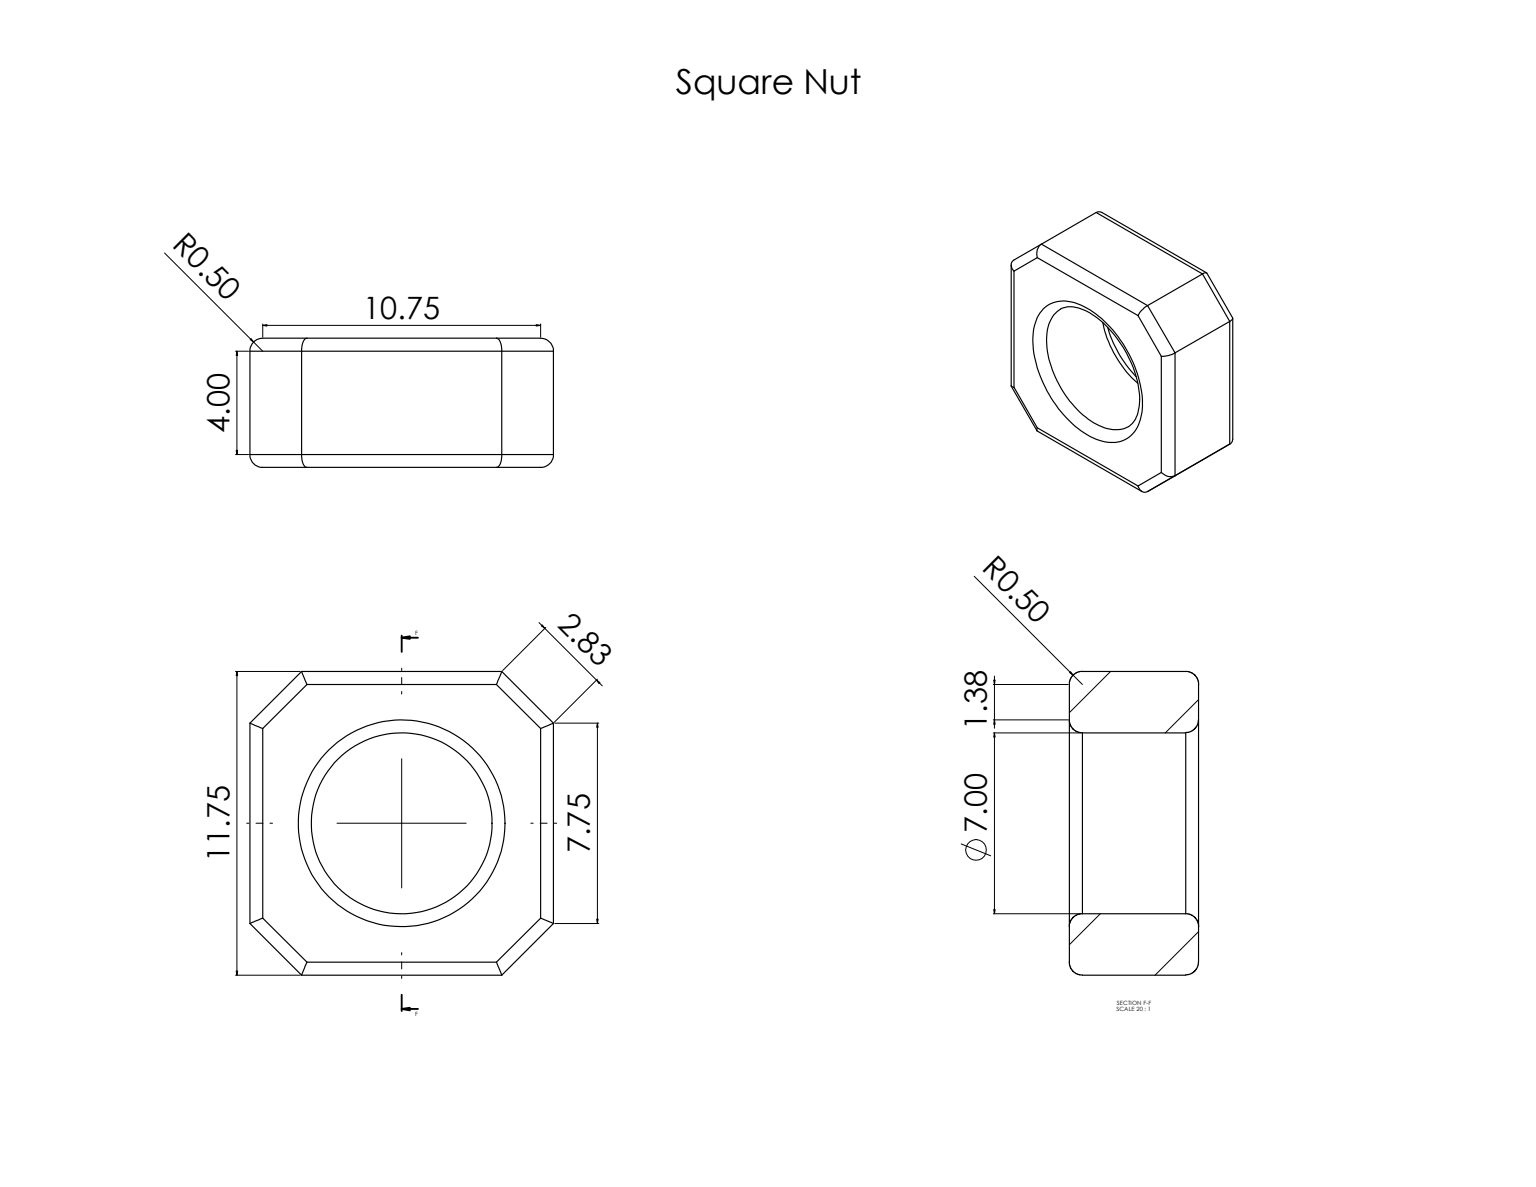
ISO-10303-21;
HEADER;
FILE_DESCRIPTION (('STEP AP214'),
    '1' );
FILE_NAME ('Square Nut.step',
    '2026-10-25T21:42:00',
    ( '' ),
    ( '' ),
    'SwSTEP 2.0',
    'SolidWorks 2025',
    '' );
FILE_SCHEMA (( 'AUTOMOTIVE_DESIGN' ));
ENDSEC;

DATA;
#32=VECTOR ( 'NONE', #10957, 1000.000000000000000 ) ;
#147=EDGE_LOOP ( 'NONE', ( #29391, #20938, #24659, #15667, #28706, #3873, #20369, #28509 ) ) ;
#209=ORIENTED_EDGE ( 'NONE', *, *, #21676, .F. ) ;
#298=LINE ( 'NONE', #12862, #20525 ) ;
#314=ORIENTED_EDGE ( 'NONE', *, *, #36050, .T. ) ;
#343=VECTOR ( 'NONE', #5203, 999.9999999999998863 ) ;
#423=ORIENTED_EDGE ( 'NONE', *, *, #22211, .T. ) ;
#429=CARTESIAN_POINT ( 'NONE',  ( 0.000000000000000000, 17.49999999999998934, -84.65254291642213502 ) ) ;
#439=EDGE_CURVE ( 'NONE', #4506, #37991, #39370, .T. ) ;
#451=( NAMED_UNIT ( * ) PLANE_ANGLE_UNIT ( ) SI_UNIT ( $, .RADIAN. ) );
#460=DIRECTION ( 'NONE',  ( 1.000000000000000000, 0.000000000000000000, 0.000000000000000000 ) ) ;
#514=EDGE_CURVE ( 'NONE', #7458, #11015, #14082, .T. ) ;
#541=ADVANCED_FACE ( 'NONE', ( #26216 ), #32999, .F. ) ;
#599=VECTOR ( 'NONE', #23370, 1000.000000000000000 ) ;
#676=AXIS2_PLACEMENT_3D ( 'NONE', #31077, #40644, #5545 ) ;
#731=CYLINDRICAL_SURFACE ( 'NONE', #34237, 0.5000000000000004441 ) ;
#739=ADVANCED_FACE ( 'NONE', ( #24084 ), #20878, .T. ) ;
#747=DIRECTION ( 'NONE',  ( 0.000000000000000000, -0.000000000000000000, 1.000000000000000000 ) ) ;
#835=AXIS2_PLACEMENT_3D ( 'NONE', #18209, #14814, #11404 ) ;
#865=ORIENTED_EDGE ( 'NONE', *, *, #17748, .T. ) ;
#951=PLANE ( 'NONE',  #3002 ) ;
#1004=ORIENTED_EDGE ( 'NONE', *, *, #3760, .F. ) ;
#1026=DIRECTION ( 'NONE',  ( 0.000000000000000000, 0.000000000000000000, -1.000000000000000000 ) ) ;
#1027=DIRECTION ( 'NONE',  ( -0.7071067811865469066, -0.7071067811865482389, -0.000000000000000000 ) ) ;
#1093=PLANE ( 'NONE',  #33638 ) ;
#1147=EDGE_CURVE ( 'NONE', #19379, #7458, #41009, .T. ) ;
#1148=DIRECTION ( 'NONE',  ( 0.000000000000000000, -0.000000000000000000, 1.000000000000000000 ) ) ;
#1215=CYLINDRICAL_SURFACE ( 'NONE', #6156, 0.5000000000000004441 ) ;
#1238=CYLINDRICAL_SURFACE ( 'NONE', #24874, 0.5000000000000006661 ) ;
#1268=DIRECTION ( 'NONE',  ( 0.000000000000000000, -0.000000000000000000, 1.000000000000000000 ) ) ;
#1309=CARTESIAN_POINT ( 'NONE',  ( 5.876432148649220366, 13.62356785135077075, -80.65254291642212081 ) ) ;
#1364=ORIENTED_EDGE ( 'NONE', *, *, #11107, .F. ) ;
#1384=CARTESIAN_POINT ( 'NONE',  ( -3.876432148649210152, 11.62356785135076542, -85.15254291642213502 ) ) ;
#1493=ORIENTED_EDGE ( 'NONE', *, *, #11107, .T. ) ;
#1543=ADVANCED_FACE ( 'NONE', ( #16227 ), #29170, .F. ) ;
#1548=ORIENTED_EDGE ( 'NONE', *, *, #4783, .F. ) ;
#1552=( LENGTH_UNIT ( ) NAMED_UNIT ( * ) SI_UNIT ( .MILLI., .METRE. ) );
#1590=EDGE_LOOP ( 'NONE', ( #18017, #2676, #21565, #27525 ) ) ;
#1591=CARTESIAN_POINT ( 'NONE',  ( -3.669325367462682230, 22.87643214864920438, -85.15254291642213502 ) ) ;
#1626=DIRECTION ( 'NONE',  ( 0.000000000000000000, -1.000000000000000000, 0.000000000000000000 ) ) ;
#1760=AXIS2_PLACEMENT_3D ( 'NONE', #429, #40567, #7833 ) ;
#1873=CARTESIAN_POINT ( 'NONE',  ( 0.000000000000000000, 17.49999999999998934, -84.65254291642213502 ) ) ;
#1918=CARTESIAN_POINT ( 'NONE',  ( -4.227121241944041152, 4.227121241944031382, -84.65254291642213502 ) ) ;
#1965=CARTESIAN_POINT ( 'NONE',  ( 5.876432148649220366, 13.62356785135077075, -84.65254291642213502 ) ) ;
#1990=ORIENTED_EDGE ( 'NONE', *, *, #41545, .T. ) ;
#1995=( BOUNDED_CURVE ( )  B_SPLINE_CURVE ( 3, ( #10609, #7625, #33578, #29950 ),
 .UNSPECIFIED., .F., .T. ) 
 B_SPLINE_CURVE_WITH_KNOTS ( ( 4, 4 ),
 ( 4.712388980384687009, 6.283185307179586232 ),
 .UNSPECIFIED. ) 
 CURVE ( )  GEOMETRIC_REPRESENTATION_ITEM ( )  RATIONAL_B_SPLINE_CURVE ( ( 1.000000000000000000, 0.8047378541243643824, 0.8047378541243643824, 1.000000000000000000 ) ) 
 REPRESENTATION_ITEM ( '' )  );
#1996=ORIENTED_EDGE ( 'NONE', *, *, #24896, .F. ) ;
#2058=VECTOR ( 'NONE', #38392, 1000.000000000000114 ) ;
#2077=CARTESIAN_POINT ( 'NONE',  ( -3.876432148649222142, 23.37643214864920438, -84.65254291642213502 ) ) ;
#2139=ORIENTED_EDGE ( 'NONE', *, *, #24461, .F. ) ;
#2181=DIRECTION ( 'NONE',  ( -0.7071067811865491270, 0.7071067811865460184, 0.000000000000000000 ) ) ;
#2237=CARTESIAN_POINT ( 'NONE',  ( 5.876432148649220366, 21.37643214864921148, -84.65254291642213502 ) ) ;
#2249=FACE_OUTER_BOUND ( 'NONE', #36965, .T. ) ;
#2266=CARTESIAN_POINT ( 'NONE',  ( 3.876432148649220366, 11.62356785135076542, -80.65254291642212081 ) ) ;
#2363=EDGE_LOOP ( 'NONE', ( #33667, #25250 ) ) ;
#2397=TOROIDAL_SURFACE ( 'NONE', #13937, 4.000000000000003553, 0.5000000000000000000 ) ;
#2455=VERTEX_POINT ( 'NONE', #23151 ) ;
#2474=ORIENTED_EDGE ( 'NONE', *, *, #36963, .T. ) ;
#2499=FACE_OUTER_BOUND ( 'NONE', #41086, .T. ) ;
#2517=ADVANCED_FACE ( 'NONE', ( #16367 ), #9981, .F. ) ;
#2561=ORIENTED_EDGE ( 'NONE', *, *, #32470, .T. ) ;
#2601=ORIENTED_EDGE ( 'NONE', *, *, #36050, .F. ) ;
#2676=ORIENTED_EDGE ( 'NONE', *, *, #13612, .F. ) ;
#2698=AXIS2_PLACEMENT_3D ( 'NONE', #15484, #25686, #38648 ) ;
#2718=DIRECTION ( 'NONE',  ( -0.7071067811865465735, -0.7071067811865483499, -0.000000000000000000 ) ) ;
#2762=DIRECTION ( 'NONE',  ( 0.7071067811865490160, -0.7071067811865460184, -0.000000000000000000 ) ) ;
#2811=DIRECTION ( 'NONE',  ( 0.000000000000000000, 0.000000000000000000, -1.000000000000000000 ) ) ;
#2845=EDGE_CURVE ( 'NONE', #19607, #21730, #21811, .T. ) ;
#2917=CARTESIAN_POINT ( 'NONE',  ( 3.669325367462673793, 12.12356785135076542, -80.15254291642212081 ) ) ;
#2983=ORIENTED_EDGE ( 'NONE', *, *, #7409, .T. ) ;
#3002=AXIS2_PLACEMENT_3D ( 'NONE', #30076, #23711, #13917 ) ;
#3094=ADVANCED_FACE ( 'NONE', ( #32468 ), #36285, .T. ) ;
#3161=ORIENTED_EDGE ( 'NONE', *, *, #23680, .T. ) ;
#3163=VECTOR ( 'NONE', #21410, 1000.000000000000000 ) ;
#3352=DIRECTION ( 'NONE',  ( -1.000000000000000000, -0.000000000000000000, -0.000000000000000000 ) ) ;
#3399=ORIENTED_EDGE ( 'NONE', *, *, #5823, .T. ) ;
#3527=DIRECTION ( 'NONE',  ( 1.000000000000000000, 0.000000000000000000, -0.000000000000000000 ) ) ;
#3569=AXIS2_PLACEMENT_3D ( 'NONE', #31939, #13418, #2811 ) ;
#3608=ADVANCED_FACE ( 'NONE', ( #17255 ), #1093, .F. ) ;
#3668=VERTEX_POINT ( 'NONE', #26610 ) ;
#3679=AXIS2_PLACEMENT_3D ( 'NONE', #26780, #39745, #29310 ) ;
#3745=CARTESIAN_POINT ( 'NONE',  ( -4.227121241944041152, 4.227121241944031382, -80.65254291642212081 ) ) ;
#3760=EDGE_CURVE ( 'NONE', #27278, #9802, #11736, .T. ) ;
#3765=CARTESIAN_POINT ( 'NONE',  ( -5.876432148649216813, 13.62356785135076365, -80.35964969760868826 ) ) ;
#3777=AXIS2_PLACEMENT_3D ( 'NONE', #10554, #23535, #36496 ) ;
#3816=CARTESIAN_POINT ( 'NONE',  ( 5.376432148649220366, 11.62356785135076542, -80.65254291642212081 ) ) ;
#3840=ORIENTED_EDGE ( 'NONE', *, *, #23636, .T. ) ;
#3856=DIRECTION ( 'NONE',  ( 1.000000000000000000, 0.000000000000000000, 0.000000000000000000 ) ) ;
#3873=ORIENTED_EDGE ( 'NONE', *, *, #4783, .T. ) ;
#3931=EDGE_LOOP ( 'NONE', ( #11008, #40649, #40449, #39510 ) ) ;
#4095=CARTESIAN_POINT ( 'NONE',  ( -5.669325367462669796, 13.70935428897766428, -85.15254291642212081 ) ) ;
#4249=AXIS2_PLACEMENT_3D ( 'NONE', #22294, #5923, #12518 ) ;
#4280=CARTESIAN_POINT ( 'NONE',  ( 0.000000000000000000, 17.49999999999998934, -80.65254291642212081 ) ) ;
#4479=ORIENTED_EDGE ( 'NONE', *, *, #27721, .F. ) ;
#4506=VERTEX_POINT ( 'NONE', #29675 ) ;
#4555=CYLINDRICAL_SURFACE ( 'NONE', #36145, 0.5000000000000000000 ) ;
#4624=VERTEX_POINT ( 'NONE', #17969 ) ;
#4632=CARTESIAN_POINT ( 'NONE',  ( -13.27287875805594375, 13.27287875805592243, -84.65254291642213502 ) ) ;
#4703=DIRECTION ( 'NONE',  ( -0.7071067811865466846, -0.7071067811865484609, 0.000000000000000000 ) ) ;
#4721=VECTOR ( 'NONE', #40569, 1000.000000000000000 ) ;
#4727=CARTESIAN_POINT ( 'NONE',  ( -3.876432148649210152, 11.62356785135076542, -84.65254291642213502 ) ) ;
#4758=ORIENTED_EDGE ( 'NONE', *, *, #23038, .F. ) ;
#4783=EDGE_CURVE ( 'NONE', #32392, #14391, #31561, .T. ) ;
#4794=AXIS2_PLACEMENT_3D ( 'NONE', #22231, #12453, #15231 ) ;
#4816=CARTESIAN_POINT ( 'NONE',  ( 5.376432148649220366, 21.37643214864921148, -80.15254291642212081 ) ) ;
#4832=LINE ( 'NONE', #17809, #16083 ) ;
#4930=DIRECTION ( 'NONE',  ( 1.224646799147353207E-16, 1.000000000000000000, 0.000000000000000000 ) ) ;
#4940=EDGE_LOOP ( 'NONE', ( #39227, #40543, #33166, #21180 ) ) ;
#4991=VECTOR ( 'NONE', #23873, 1000.000000000000000 ) ;
#5078=CARTESIAN_POINT ( 'NONE',  ( 5.876432148649220366, 13.62356785135077075, -80.65254291642212081 ) ) ;
#5130=ORIENTED_EDGE ( 'NONE', *, *, #17603, .F. ) ;
#5166=CARTESIAN_POINT ( 'NONE',  ( 5.376432148649220366, 13.83067463253731688, -85.15254291642213502 ) ) ;
#5199=DIRECTION ( 'NONE',  ( 1.000000000000000000, 0.000000000000000000, 0.000000000000000000 ) ) ;
#5203=DIRECTION ( 'NONE',  ( 0.7071067811865469066, 0.7071067811865482389, -0.000000000000000000 ) ) ;
#5251=VERTEX_POINT ( 'NONE', #7602 ) ;
#5280=LINE ( 'NONE', #40592, #16563 ) ;
#5325=DIRECTION ( 'NONE',  ( 0.000000000000000000, -1.000000000000000000, 0.000000000000000000 ) ) ;
#5458=CARTESIAN_POINT ( 'NONE',  ( 5.876432148649220366, 11.62356785135076542, -84.65254291642213502 ) ) ;
#5482=CARTESIAN_POINT ( 'NONE',  ( 3.876432148649219034, 23.37643214864920438, -80.35964969760868826 ) ) ;
#5545=DIRECTION ( 'NONE',  ( 0.000000000000000000, 0.000000000000000000, 1.000000000000000000 ) ) ;
#5580=VECTOR ( 'NONE', #3352, 1000.000000000000000 ) ;
#5674=ORIENTED_EDGE ( 'NONE', *, *, #23056, .T. ) ;
#5718=ORIENTED_EDGE ( 'NONE', *, *, #24896, .T. ) ;
#5753=CARTESIAN_POINT ( 'NONE',  ( 0.000000000000000000, 12.12356785135076542, -85.15254291642213502 ) ) ;
#5823=EDGE_CURVE ( 'NONE', #5925, #2455, #7405, .T. ) ;
#5876=ORIENTED_EDGE ( 'NONE', *, *, #10287, .T. ) ;
#5892=UNCERTAINTY_MEASURE_WITH_UNIT (LENGTH_MEASURE( 1.000000000000000082E-05 ), #1552, 'distance_accuracy_value', 'NONE');
#5923=DIRECTION ( 'NONE',  ( 0.000000000000000000, 1.000000000000000000, 0.000000000000000000 ) ) ;
#5925=VERTEX_POINT ( 'NONE', #32155 ) ;
#5973=APPLICATION_CONTEXT ( 'automotive_design' ) ;
#5979=EDGE_LOOP ( 'NONE', ( #31636, #15185, #4479, #36051 ) ) ;
#6042=DIRECTION ( 'NONE',  ( 0.7071067811865493491, -0.7071067811865456854, -0.000000000000000000 ) ) ;
#6082=ADVANCED_FACE ( 'NONE', ( #6418 ), #26203, .T. ) ;
#6156=AXIS2_PLACEMENT_3D ( 'NONE', #26955, #1626, #37356 ) ;
#6175=EDGE_LOOP ( 'NONE', ( #38409, #6967, #1004, #22355 ) ) ;
#6180=EDGE_LOOP ( 'NONE', ( #37873, #40148, #25285, #33874 ) ) ;
#6286=ORIENTED_EDGE ( 'NONE', *, *, #34782, .F. ) ;
#6404=ORIENTED_EDGE ( 'NONE', *, *, #36318, .T. ) ;
#6418=FACE_OUTER_BOUND ( 'NONE', #6180, .T. ) ;
#6461=CARTESIAN_POINT ( 'NONE',  ( -5.376432148649216813, 21.16932536746266891, -85.15254291642213502 ) ) ;
#6492=FACE_OUTER_BOUND ( 'NONE', #31237, .T. ) ;
#6540=ADVANCED_FACE ( 'NONE', ( #34043 ), #30853, .F. ) ;
#6601=ORIENTED_EDGE ( 'NONE', *, *, #3760, .T. ) ;
#6722=PRODUCT_DEFINITION_CONTEXT ( 'detailed design', #34229, 'design' ) ;
#6755=CARTESIAN_POINT ( 'NONE',  ( -3.876432148649210152, 11.62356785135076542, -80.65254291642212081 ) ) ;
#6841=CARTESIAN_POINT ( 'NONE',  ( 0.000000000000000000, 17.49999999999998934, -85.15254291642213502 ) ) ;
#6869=CARTESIAN_POINT ( 'NONE',  ( 3.876432148649218590, 23.37643214864920438, -84.65254291642213502 ) ) ;
#6933=DIRECTION ( 'NONE',  ( 0.000000000000000000, -0.000000000000000000, 1.000000000000000000 ) ) ;
#6967=ORIENTED_EDGE ( 'NONE', *, *, #7673, .F. ) ;
#6984=EDGE_CURVE ( 'NONE', #15190, #40136, #40460, .T. ) ;
#6988=DIRECTION ( 'NONE',  ( -0.7071067811865493491, 0.7071067811865456854, 0.000000000000000000 ) ) ;
#7018=VERTEX_POINT ( 'NONE', #31120 ) ;
#7026=VECTOR ( 'NONE', #10044, 1000.000000000000000 ) ;
#7045=( NAMED_UNIT ( * ) SI_UNIT ( $, .STERADIAN. ) SOLID_ANGLE_UNIT ( ) );
#7059=VECTOR ( 'NONE', #39067, 1000.000000000000000 ) ;
#7092=( BOUNDED_CURVE ( )  B_SPLINE_CURVE ( 3, ( #6755, #38245, #19728, #32697 ),
 .UNSPECIFIED., .F., .T. ) 
 B_SPLINE_CURVE_WITH_KNOTS ( ( 4, 4 ),
 ( 3.141592653589793116, 4.712388980384691450 ),
 .UNSPECIFIED. ) 
 CURVE ( )  GEOMETRIC_REPRESENTATION_ITEM ( )  RATIONAL_B_SPLINE_CURVE ( ( 1.000000000000000000, 0.8047378541243646044, 0.8047378541243646044, 1.000000000000000000 ) ) 
 REPRESENTATION_ITEM ( '' )  );
#7127=ORIENTED_EDGE ( 'NONE', *, *, #27437, .T. ) ;
#7129=PLANE ( 'NONE',  #23279 ) ;
#7239=ORIENTED_EDGE ( 'NONE', *, *, #32404, .T. ) ;
#7279=( BOUNDED_CURVE ( )  B_SPLINE_CURVE ( 3, ( #8666, #34617, #5482, #18458 ),
 .UNSPECIFIED., .F., .T. ) 
 B_SPLINE_CURVE_WITH_KNOTS ( ( 4, 4 ),
 ( 1.570796326794896336, 3.141592653589793116 ),
 .UNSPECIFIED. ) 
 CURVE ( )  GEOMETRIC_REPRESENTATION_ITEM ( )  RATIONAL_B_SPLINE_CURVE ( ( 1.000000000000000000, 0.8047378541243649375, 0.8047378541243649375, 1.000000000000000000 ) ) 
 REPRESENTATION_ITEM ( '' )  );
#7380=CARTESIAN_POINT ( 'NONE',  ( -5.376432148649216813, 13.83067463253730978, -80.15254291642212081 ) ) ;
#7405=( BOUNDED_CURVE ( )  B_SPLINE_CURVE ( 3, ( #5166, #15581, #34925, #1965 ),
 .UNSPECIFIED., .F., .T. ) 
 B_SPLINE_CURVE_WITH_KNOTS ( ( 4, 4 ),
 ( 4.712388980384687898, 6.283185307179586232 ),
 .UNSPECIFIED. ) 
 CURVE ( )  GEOMETRIC_REPRESENTATION_ITEM ( )  RATIONAL_B_SPLINE_CURVE ( ( 1.000000000000000000, 0.8047378541243646044, 0.8047378541243646044, 1.000000000000000000 ) ) 
 REPRESENTATION_ITEM ( '' )  );
#7409=EDGE_CURVE ( 'NONE', #7458, #7018, #22932, .T. ) ;
#7447=VECTOR ( 'NONE', #24031, 1000.000000000000114 ) ;
#7458=VERTEX_POINT ( 'NONE', #27532 ) ;
#7593=CARTESIAN_POINT ( 'NONE',  ( -5.376432148649216813, 0.000000000000000000, -85.15254291642213502 ) ) ;
#7602=CARTESIAN_POINT ( 'NONE',  ( 3.669325367462670240, 22.87643214864920438, -85.15254291642213502 ) ) ;
#7625=CARTESIAN_POINT ( 'NONE',  ( 5.669325367462671572, 21.29064571102230730, -80.15254291642210660 ) ) ;
#7673=EDGE_CURVE ( 'NONE', #9802, #11727, #25745, .T. ) ;
#7747=DIRECTION ( 'NONE',  ( 0.000000000000000000, -0.000000000000000000, 1.000000000000000000 ) ) ;
#7768=ORIENTED_EDGE ( 'NONE', *, *, #23056, .F. ) ;
#7833=DIRECTION ( 'NONE',  ( 1.000000000000000000, 0.000000000000000000, 0.000000000000000000 ) ) ;
#7975=CYLINDRICAL_SURFACE ( 'NONE', #14460, 3.500000000000003997 ) ;
#8033=DIRECTION ( 'NONE',  ( -0.7071067811865475727, 0.7071067811865475727, 0.000000000000000000 ) ) ;
#8121=FACE_OUTER_BOUND ( 'NONE', #20680, .T. ) ;
#8235=CARTESIAN_POINT ( 'NONE',  ( 3.876432148649220366, 11.62356785135076542, -85.15254291642213502 ) ) ;
#8279=ORIENTED_EDGE ( 'NONE', *, *, #439, .F. ) ;
#8374=VERTEX_POINT ( 'NONE', #10158 ) ;
#8499=EDGE_CURVE ( 'NONE', #24919, #18881, #13981, .T. ) ;
#8552=VECTOR ( 'NONE', #14206, 1000.000000000000000 ) ;
#8597=CARTESIAN_POINT ( 'NONE',  ( 5.376432148649219478, 21.16932536746266535, -85.15254291642213502 ) ) ;
#8641=ORIENTED_EDGE ( 'NONE', *, *, #15208, .F. ) ;
#8665=PLANE ( 'NONE',  #2698 ) ;
#8666=CARTESIAN_POINT ( 'NONE',  ( 3.669325367462669796, 22.87643214864920438, -80.15254291642212081 ) ) ;
#8871=AXIS2_PLACEMENT_3D ( 'NONE', #25817, #19834, #32595 ) ;
#8876=CARTESIAN_POINT ( 'NONE',  ( 3.876432148649220366, 11.62356785135076542, -80.65254291642212081 ) ) ;
#8889=DIRECTION ( 'NONE',  ( -0.000000000000000000, -0.000000000000000000, 1.000000000000000000 ) ) ;
#9049=CYLINDRICAL_SURFACE ( 'NONE', #4794, 0.4999999999999994449 ) ;
#9059=EDGE_LOOP ( 'NONE', ( #3399, #37975, #6601, #27316 ) ) ;
#9152=FACE_OUTER_BOUND ( 'NONE', #13339, .T. ) ;
#9161=VECTOR ( 'NONE', #39294, 1000.000000000000000 ) ;
#9205=ORIENTED_EDGE ( 'NONE', *, *, #8499, .F. ) ;
#9209=DIRECTION ( 'NONE',  ( 0.7071067811865493491, -0.7071067811865456854, -0.000000000000000000 ) ) ;
#9260=ADVANCED_FACE ( 'NONE', ( #31654 ), #21872, .T. ) ;
#9300=LINE ( 'NONE', #16528, #40870 ) ;
#9314=CARTESIAN_POINT ( 'NONE',  ( 3.522878758055947301, 11.97712124194404026, -85.15254291642213502 ) ) ;
#9326=EDGE_LOOP ( 'NONE', ( #32290, #16608, #40452, #19266 ) ) ;
#9414=CARTESIAN_POINT ( 'NONE',  ( -5.876432148649216813, 21.37643214864920438, -80.65254291642212081 ) ) ;
#9497=EDGE_CURVE ( 'NONE', #15673, #4506, #32725, .T. ) ;
#9608=TOROIDAL_SURFACE ( 'NONE', #19772, 4.000000000000003553, 0.5000000000000000000 ) ;
#9652=FACE_OUTER_BOUND ( 'NONE', #6175, .T. ) ;
#9659=VECTOR ( 'NONE', #1026, 1000.000000000000000 ) ;
#9660=CARTESIAN_POINT ( 'NONE',  ( 3.876432148649217257, 23.37643214864920438, -84.94543613523558179 ) ) ;
#9766=AXIS2_PLACEMENT_3D ( 'NONE', #40391, #1268, #14236 ) ;
#9802=VERTEX_POINT ( 'NONE', #11142 ) ;
#9861=ADVANCED_FACE ( 'NONE', ( #14544 ), #10927, .T. ) ;
#9921=DIRECTION ( 'NONE',  ( 0.000000000000000000, -0.000000000000000000, 1.000000000000000000 ) ) ;
#9937=AXIS2_PLACEMENT_3D ( 'NONE', #41835, #31405, #24620 ) ;
#9952=CARTESIAN_POINT ( 'NONE',  ( -5.876432148649216813, 21.37643214864920438, -80.65254291642212081 ) ) ;
#9953=ORIENTED_EDGE ( 'NONE', *, *, #12643, .T. ) ;
#9981=PLANE ( 'NONE',  #3679 ) ;
#9994=CARTESIAN_POINT ( 'NONE',  ( 0.000000000000000000, 17.49999999999998934, -84.65254291642213502 ) ) ;
#10044=DIRECTION ( 'NONE',  ( 1.000000000000000000, 0.000000000000000000, 0.000000000000000000 ) ) ;
#10046=EDGE_LOOP ( 'NONE', ( #25900, #18008, #20047, #1990 ) ) ;
#10135=CARTESIAN_POINT ( 'NONE',  ( -3.669325367462664911, 12.12356785135076542, -85.15254291642213502 ) ) ;
#10158=CARTESIAN_POINT ( 'NONE',  ( -3.500000000000003997, 17.49999999999998934, -84.65254291642213502 ) ) ;
#10193=MANIFOLD_SOLID_BREP ( 'Body-Move/Copy2', #41675 ) ;
#10208=ORIENTED_EDGE ( 'NONE', *, *, #32404, .F. ) ;
#10287=EDGE_CURVE ( 'NONE', #18881, #40136, #38916, .T. ) ;
#10296=CARTESIAN_POINT ( 'NONE',  ( 3.876432148649218590, 23.37643214864920438, -85.15254291642213502 ) ) ;
#10382=SHAPE_REPRESENTATION ( 'Square Nut', ( #40442 ), #22097 ) ;
#10446=DIRECTION ( 'NONE',  ( 0.000000000000000000, 0.000000000000000000, 1.000000000000000000 ) ) ;
#10530=VERTEX_POINT ( 'NONE', #18921 ) ;
#10540=SHAPE_DEFINITION_REPRESENTATION ( #17341, #10382 ) ;
#10554=CARTESIAN_POINT ( 'NONE',  ( -4.000000000000003553, 17.49999999999998934, -80.65254291642212081 ) ) ;
#10598=LINE ( 'NONE', #10798, #34394 ) ;
#10609=CARTESIAN_POINT ( 'NONE',  ( 5.376432148649220366, 21.16932536746266180, -80.15254291642212081 ) ) ;
#10646=DIRECTION ( 'NONE',  ( 0.7071067811865469066, 0.7071067811865482389, -0.000000000000000000 ) ) ;
#10671=FACE_OUTER_BOUND ( 'NONE', #9059, .T. ) ;
#10722=DIRECTION ( 'NONE',  ( -0.7071067811865459074, -0.7071067811865493491, 0.000000000000000000 ) ) ;
#10788=ORIENTED_EDGE ( 'NONE', *, *, #10287, .F. ) ;
#10798=CARTESIAN_POINT ( 'NONE',  ( -13.27287875805594375, 13.27287875805592243, -80.15254291642212081 ) ) ;
#10804=DIRECTION ( 'NONE',  ( 1.000000000000000000, 0.000000000000000000, 0.000000000000000000 ) ) ;
#10888=CARTESIAN_POINT ( 'NONE',  ( -5.876432148649216813, 21.37643214864920438, -85.15254291642213502 ) ) ;
#10905=AXIS2_PLACEMENT_3D ( 'NONE', #14550, #7747, #27314 ) ;
#10927=CYLINDRICAL_SURFACE ( 'NONE', #13751, 0.5000000000000000000 ) ;
#10957=DIRECTION ( 'NONE',  ( 0.000000000000000000, 0.000000000000000000, -1.000000000000000000 ) ) ;
#10961=ORIENTED_EDGE ( 'NONE', *, *, #38240, .F. ) ;
#11008=ORIENTED_EDGE ( 'NONE', *, *, #24661, .T. ) ;
#11015=VERTEX_POINT ( 'NONE', #17218 ) ;
#11058=STYLED_ITEM('',(#42159),#10193);
#11065=EDGE_CURVE ( 'NONE', #5925, #9802, #34836, .T. ) ;
#11078=VECTOR ( 'NONE', #2718, 1000.000000000000114 ) ;
#11102=EDGE_LOOP ( 'NONE', ( #865, #423 ) ) ;
#11107=EDGE_CURVE ( 'NONE', #8374, #40136, #38026, .T. ) ;
#11131=CARTESIAN_POINT ( 'NONE',  ( 0.000000000000000000, 0.000000000000000000, 0.000000000000000000 ) ) ;
#11142=CARTESIAN_POINT ( 'NONE',  ( 3.669325367462672904, 12.12356785135076542, -85.15254291642213502 ) ) ;
#11174=ORIENTED_EDGE ( 'NONE', *, *, #38240, .T. ) ;
#11202=ORIENTED_EDGE ( 'NONE', *, *, #20692, .F. ) ;
#11247=CARTESIAN_POINT ( 'NONE',  ( -3.790645711022322395, 23.16932536746265825, -85.15254291642213502 ) ) ;
#11317=CARTESIAN_POINT ( 'NONE',  ( 5.876432148649220366, 21.37643214864921148, -80.65254291642212081 ) ) ;
#11318=EDGE_CURVE ( 'NONE', #27278, #2455, #38851, .T. ) ;
#11401=EDGE_CURVE ( 'NONE', #4624, #21730, #22062, .T. ) ;
#11404=DIRECTION ( 'NONE',  ( 1.000000000000000000, 0.000000000000000000, 0.000000000000000000 ) ) ;
#11540=CARTESIAN_POINT ( 'NONE',  ( 4.227121241944058028, 4.227121241944076679, -84.65254291642213502 ) ) ;
#11573=CARTESIAN_POINT ( 'NONE',  ( -3.522878758055951298, 23.02287875805593487, -85.15254291642213502 ) ) ;
#11612=ORIENTED_EDGE ( 'NONE', *, *, #22194, .T. ) ;
#11727=VERTEX_POINT ( 'NONE', #10135 ) ;
#11736=( BOUNDED_CURVE ( )  B_SPLINE_CURVE ( 3, ( #17671, #27856, #17875, #15102 ),
 .UNSPECIFIED., .F., .T. ) 
 B_SPLINE_CURVE_WITH_KNOTS ( ( 4, 4 ),
 ( 3.141592653589793116, 4.712388980384693227 ),
 .UNSPECIFIED. ) 
 CURVE ( )  GEOMETRIC_REPRESENTATION_ITEM ( )  RATIONAL_B_SPLINE_CURVE ( ( 1.000000000000000000, 0.8047378541243641603, 0.8047378541243641603, 1.000000000000000000 ) ) 
 REPRESENTATION_ITEM ( '' )  );
#11825=EDGE_LOOP ( 'NONE', ( #1364, #3840, #15028, #5876 ) ) ;
#11831=DIRECTION ( 'NONE',  ( -0.7071067811865465735, -0.7071067811865483499, 0.000000000000000000 ) ) ;
#11866=CARTESIAN_POINT ( 'NONE',  ( -4.000000000000003553, 17.49999999999998934, -85.15254291642213502 ) ) ;
#11884=CARTESIAN_POINT ( 'NONE',  ( -3.669325367462680010, 22.87643214864920438, -80.15254291642212081 ) ) ;
#12132=VECTOR ( 'NONE', #6988, 1000.000000000000000 ) ;
#12267=TOROIDAL_SURFACE ( 'NONE', #15015, 4.000000000000003553, 0.5000000000000000000 ) ;
#12304=LINE ( 'NONE', #38043, #41884 ) ;
#12312=ADVANCED_FACE ( 'NONE', ( #28916 ), #32112, .T. ) ;
#12388=ORIENTED_EDGE ( 'NONE', *, *, #21315, .F. ) ;
#12426=FACE_OUTER_BOUND ( 'NONE', #20888, .T. ) ;
#12453=DIRECTION ( 'NONE',  ( 0.7071067811865493491, -0.7071067811865456854, -0.000000000000000000 ) ) ;
#12508=ADVANCED_FACE ( 'NONE', ( #29547 ), #13388, .T. ) ;
#12518=DIRECTION ( 'NONE',  ( 0.000000000000000000, 0.000000000000000000, 1.000000000000000000 ) ) ;
#12638=CARTESIAN_POINT ( 'NONE',  ( 13.27287875805592776, 13.27287875805599704, -84.65254291642213502 ) ) ;
#12643=EDGE_CURVE ( 'NONE', #16965, #39500, #22709, .T. ) ;
#12644=CARTESIAN_POINT ( 'NONE',  ( -5.876432148649216813, 13.62356785135076365, -80.65254291642212081 ) ) ;
#12778=ORIENTED_EDGE ( 'NONE', *, *, #25173, .F. ) ;
#12783=ADVANCED_FACE ( 'NONE', ( #32283 ), #4555, .T. ) ;
#12811=( BOUNDED_CURVE ( )  B_SPLINE_CURVE ( 3, ( #41236, #31231, #37414, #5078 ),
 .UNSPECIFIED., .F., .T. ) 
 B_SPLINE_CURVE_WITH_KNOTS ( ( 4, 4 ),
 ( 1.570796326794896558, 3.141592653589793116 ),
 .UNSPECIFIED. ) 
 CURVE ( )  GEOMETRIC_REPRESENTATION_ITEM ( )  RATIONAL_B_SPLINE_CURVE ( ( 1.000000000000000000, 0.8047378541243649375, 0.8047378541243649375, 1.000000000000000000 ) ) 
 REPRESENTATION_ITEM ( '' )  );
#12853=AXIS2_PLACEMENT_3D ( 'NONE', #17816, #20593, #10804 ) ;
#12862=CARTESIAN_POINT ( 'NONE',  ( -5.522878758055947301, 13.97712124194404026, -85.15254291642213502 ) ) ;
#12887=ORIENTED_EDGE ( 'NONE', *, *, #17748, .F. ) ;
#12888=FACE_BOUND ( 'NONE', #2363, .T. ) ;
#13049=CARTESIAN_POINT ( 'NONE',  ( -5.876432148649216813, 21.37643214864920438, -84.65254291642213502 ) ) ;
#13069=LINE ( 'NONE', #10296, #15646 ) ;
#13087=ORIENTED_EDGE ( 'NONE', *, *, #25343, .F. ) ;
#13111=UNCERTAINTY_MEASURE_WITH_UNIT (LENGTH_MEASURE( 1.000000000000000082E-05 ), #20024, 'distance_accuracy_value', 'NONE');
#13117=DIRECTION ( 'NONE',  ( -0.7071067811865466846, -0.7071067811865484609, 0.000000000000000000 ) ) ;
#13222=DIRECTION ( 'NONE',  ( 0.000000000000000000, -0.000000000000000000, 1.000000000000000000 ) ) ;
#13252=CYLINDRICAL_SURFACE ( 'NONE', #8871, 0.5000000000000004441 ) ;
#13301=ORIENTED_EDGE ( 'NONE', *, *, #9497, .T. ) ;
#13321=CIRCLE ( 'NONE', #1760, 3.500000000000003997 ) ;
#13339=EDGE_LOOP ( 'NONE', ( #23450, #38683, #31091, #7239 ) ) ;
#13355=CARTESIAN_POINT ( 'NONE',  ( -3.669325367462680010, 22.87643214864920438, -80.15254291642212081 ) ) ;
#13357=ORIENTED_EDGE ( 'NONE', *, *, #2845, .T. ) ;
#13388=CYLINDRICAL_SURFACE ( 'NONE', #25288, 0.5000000000000004441 ) ;
#13401=LINE ( 'NONE', #8235, #8552 ) ;
#13418=DIRECTION ( 'NONE',  ( 0.000000000000000000, -1.000000000000000000, 0.000000000000000000 ) ) ;
#13435=EDGE_CURVE ( 'NONE', #17850, #3668, #19441, .T. ) ;
#13595=DIRECTION ( 'NONE',  ( 0.000000000000000000, 1.000000000000000000, 0.000000000000000000 ) ) ;
#13612=EDGE_CURVE ( 'NONE', #11727, #21607, #298, .T. ) ;
#13632=AXIS2_PLACEMENT_3D ( 'NONE', #30942, #34338, #5199 ) ;
#13724=PRODUCT_CONTEXT ( 'NONE', #5973, 'mechanical' ) ;
#13732=EDGE_CURVE ( 'NONE', #37786, #2455, #30570, .T. ) ;
#13751=AXIS2_PLACEMENT_3D ( 'NONE', #11540, #2181, #24532 ) ;
#13881=CARTESIAN_POINT ( 'NONE',  ( -3.790645711022310405, 11.83067463253731688, -85.15254291642212081 ) ) ;
#13917=DIRECTION ( 'NONE',  ( 0.000000000000000000, 0.000000000000000000, 1.000000000000000000 ) ) ;
#13930=EDGE_LOOP ( 'NONE', ( #4758, #15612, #39324, #1548 ) ) ;
#13937=AXIS2_PLACEMENT_3D ( 'NONE', #30275, #1148, #14116 ) ;
#13981=LINE ( 'NONE', #33547, #36832 ) ;
#14041=VECTOR ( 'NONE', #11831, 1000.000000000000114 ) ;
#14064=CARTESIAN_POINT ( 'NONE',  ( -3.876432148649222142, 23.37643214864920438, -85.15254291642213502 ) ) ;
#14082=LINE ( 'NONE', #10888, #4991 ) ;
#14101=LINE ( 'NONE', #27074, #18472 ) ;
#14102=CARTESIAN_POINT ( 'NONE',  ( -5.376432148649216813, 13.83067463253730978, -85.15254291642213502 ) ) ;
#14116=DIRECTION ( 'NONE',  ( 1.000000000000000000, 0.000000000000000000, 0.000000000000000000 ) ) ;
#14183=ADVANCED_FACE ( 'NONE', ( #12888, #25867 ), #7129, .F. ) ;
#14206=DIRECTION ( 'NONE',  ( 0.000000000000000000, 0.000000000000000000, 1.000000000000000000 ) ) ;
#14236=DIRECTION ( 'NONE',  ( 1.000000000000000000, 0.000000000000000000, 0.000000000000000000 ) ) ;
#14391=VERTEX_POINT ( 'NONE', #1591 ) ;
#14411=CIRCLE ( 'NONE', #835, 4.000000000000003553 ) ;
#14455=ADVANCED_FACE ( 'NONE', ( #27118 ), #7975, .F. ) ;
#14460=AXIS2_PLACEMENT_3D ( 'NONE', #23939, #33278, #20943 ) ;
#14501=DIRECTION ( 'NONE',  ( 0.000000000000000000, 0.000000000000000000, 1.000000000000000000 ) ) ;
#14544=FACE_OUTER_BOUND ( 'NONE', #1590, .T. ) ;
#14550=CARTESIAN_POINT ( 'NONE',  ( 0.000000000000000000, 17.49999999999998934, -85.15254291642213502 ) ) ;
#14813=EDGE_CURVE ( 'NONE', #18428, #11727, #35218, .T. ) ;
#14814=DIRECTION ( 'NONE',  ( 0.000000000000000000, -0.000000000000000000, 1.000000000000000000 ) ) ;
#14850=LINE ( 'NONE', #24641, #24845 ) ;
#14854=DIRECTION ( 'NONE',  ( 1.000000000000000000, 0.000000000000000000, 0.000000000000000000 ) ) ;
#15006=CARTESIAN_POINT ( 'NONE',  ( 5.669325367462672460, 21.29064571102231795, -85.15254291642212081 ) ) ;
#15015=AXIS2_PLACEMENT_3D ( 'NONE', #19894, #9921, #38626 ) ;
#15028=ORIENTED_EDGE ( 'NONE', *, *, #8499, .T. ) ;
#15032=EDGE_LOOP ( 'NONE', ( #314, #1493, #11174, #9205 ) ) ;
#15046=EDGE_CURVE ( 'NONE', #14391, #5251, #41510, .T. ) ;
#15102=CARTESIAN_POINT ( 'NONE',  ( 3.669325367462672904, 12.12356785135076542, -85.15254291642213502 ) ) ;
#15131=ORIENTED_EDGE ( 'NONE', *, *, #15462, .F. ) ;
#15148=CIRCLE ( 'NONE', #21275, 0.5000000000000004441 ) ;
#15185=ORIENTED_EDGE ( 'NONE', *, *, #15208, .T. ) ;
#15190=VERTEX_POINT ( 'NONE', #27895 ) ;
#15208=EDGE_CURVE ( 'NONE', #8374, #38251, #15148, .T. ) ;
#15231=DIRECTION ( 'NONE',  ( 0.7071067811865457964, 0.7071067811865492381, 0.000000000000000000 ) ) ;
#15421=FACE_OUTER_BOUND ( 'NONE', #24496, .T. ) ;
#15462=EDGE_CURVE ( 'NONE', #7458, #4506, #15772, .T. ) ;
#15484=CARTESIAN_POINT ( 'NONE',  ( -5.876432148649216813, 13.62356785135076365, -85.15254291642213502 ) ) ;
#15581=CARTESIAN_POINT ( 'NONE',  ( 5.669325367462672460, 13.70935428897767672, -85.15254291642212081 ) ) ;
#15612=ORIENTED_EDGE ( 'NONE', *, *, #25282, .F. ) ;
#15646=VECTOR ( 'NONE', #26465, 1000.000000000000000 ) ;
#15667=ORIENTED_EDGE ( 'NONE', *, *, #13612, .T. ) ;
#15673=VERTEX_POINT ( 'NONE', #11884 ) ;
#15688=DIRECTION ( 'NONE',  ( 0.7071067811865465735, 0.7071067811865483499, -0.000000000000000000 ) ) ;
#15747=DIRECTION ( 'NONE',  ( 0.000000000000000000, -0.000000000000000000, 1.000000000000000000 ) ) ;
#15772=LINE ( 'NONE', #39553, #24004 ) ;
#15919=CARTESIAN_POINT ( 'NONE',  ( -3.500000000000003997, 17.49999999999998934, -85.15254291642213502 ) ) ;
#16000=ORIENTED_EDGE ( 'NONE', *, *, #11401, .F. ) ;
#16052=CARTESIAN_POINT ( 'NONE',  ( -5.669325367462668019, 21.29064571102231085, -85.15254291642214923 ) ) ;
#16053=CARTESIAN_POINT ( 'NONE',  ( 5.376432148649220366, 13.83067463253731688, -80.15254291642212081 ) ) ;
#16083=VECTOR ( 'NONE', #21205, 1000.000000000000000 ) ;
#16139=DIRECTION ( 'NONE',  ( -0.7071067811865475727, 0.7071067811865475727, 0.000000000000000000 ) ) ;
#16161=CARTESIAN_POINT ( 'NONE',  ( -5.376432148649216813, 21.16932536746266891, -85.15254291642213502 ) ) ;
#16227=FACE_OUTER_BOUND ( 'NONE', #9326, .T. ) ;
#16287=VECTOR ( 'NONE', #32956, 1000.000000000000000 ) ;
#16367=FACE_OUTER_BOUND ( 'NONE', #30989, .T. ) ;
#16384=DIRECTION ( 'NONE',  ( 1.000000000000000000, 0.000000000000000000, -0.000000000000000000 ) ) ;
#16401=ADVANCED_FACE ( 'NONE', ( #8121 ), #34483, .F. ) ;
#16443=VECTOR ( 'NONE', #20568, 1000.000000000000000 ) ;
#16521=VECTOR ( 'NONE', #24509, 1000.000000000000000 ) ;
#16528=CARTESIAN_POINT ( 'NONE',  ( -5.876432148649216813, 11.62356785135076542, -84.65254291642213502 ) ) ;
#16563=VECTOR ( 'NONE', #21033, 1000.000000000000000 ) ;
#16589=CARTESIAN_POINT ( 'NONE',  ( -5.876432148649217702, 21.37643214864920438, -84.65254291642213502 ) ) ;
#16596=ORIENTED_EDGE ( 'NONE', *, *, #25936, .F. ) ;
#16603=ORIENTED_EDGE ( 'NONE', *, *, #22194, .F. ) ;
#16608=ORIENTED_EDGE ( 'NONE', *, *, #1147, .T. ) ;
#16613=EDGE_LOOP ( 'NONE', ( #40813, #18047, #10788, #41091 ) ) ;
#16659=CARTESIAN_POINT ( 'NONE',  ( 4.000000000000003553, 17.49999999999998934, -85.15254291642213502 ) ) ;
#16686=DIRECTION ( 'NONE',  ( -0.7071067811865490160, 0.7071067811865460184, 0.000000000000000000 ) ) ;
#16749=CARTESIAN_POINT ( 'NONE',  ( -5.669325367462668908, 13.70935428897766784, -80.15254291642210660 ) ) ;
#16795=CARTESIAN_POINT ( 'NONE',  ( -4.227121241944041152, 4.227121241944031382, -80.15254291642212081 ) ) ;
#16868=CARTESIAN_POINT ( 'NONE',  ( -5.876432148649216813, 13.62356785135076365, -84.65254291642213502 ) ) ;
#16965=VERTEX_POINT ( 'NONE', #31402 ) ;
#17084=( BOUNDED_CURVE ( )  B_SPLINE_CURVE ( 3, ( #16868, #29832, #4095, #14102 ),
 .UNSPECIFIED., .F., .F. ) 
 B_SPLINE_CURVE_WITH_KNOTS ( ( 4, 4 ),
 ( 0.000000000000000000, 1.570796326794898112 ),
 .UNSPECIFIED. ) 
 CURVE ( )  GEOMETRIC_REPRESENTATION_ITEM ( )  RATIONAL_B_SPLINE_CURVE ( ( 1.000000000000000000, 0.8047378541243646044, 0.8047378541243646044, 1.000000000000000000 ) ) 
 REPRESENTATION_ITEM ( '' )  );
#17110=CARTESIAN_POINT ( 'NONE',  ( 4.227121241944058028, 4.227121241944076679, -80.65254291642212081 ) ) ;
#17112=FACE_OUTER_BOUND ( 'NONE', #10046, .T. ) ;
#17218=CARTESIAN_POINT ( 'NONE',  ( -5.876432148649216813, 21.37643214864920438, -84.65254291642213502 ) ) ;
#17255=FACE_OUTER_BOUND ( 'NONE', #27484, .T. ) ;
#17341=PRODUCT_DEFINITION_SHAPE ( 'NONE', 'NONE',  #29093 ) ;
#17360=ADVANCED_FACE ( 'NONE', ( #32448 ), #12267, .T. ) ;
#17603=EDGE_CURVE ( 'NONE', #34859, #18428, #39664, .T. ) ;
#17671=CARTESIAN_POINT ( 'NONE',  ( 3.876432148649220366, 11.62356785135076542, -84.65254291642213502 ) ) ;
#17748=EDGE_CURVE ( 'NONE', #40461, #15190, #19741, .T. ) ;
#17809=CARTESIAN_POINT ( 'NONE',  ( 5.876432148649220366, 21.37643214864921148, -85.15254291642213502 ) ) ;
#17816=CARTESIAN_POINT ( 'NONE',  ( 0.000000000000000000, 17.49999999999998934, -80.15254291642212081 ) ) ;
#17850=VERTEX_POINT ( 'NONE', #8597 ) ;
#17851=AXIS2_PLACEMENT_3D ( 'NONE', #4280, #13222, #3856 ) ;
#17875=CARTESIAN_POINT ( 'NONE',  ( 3.790645711022317066, 11.83067463253731155, -85.15254291642216344 ) ) ;
#17917=ADVANCED_FACE ( 'NONE', ( #9652 ), #13252, .T. ) ;
#17969=CARTESIAN_POINT ( 'NONE',  ( -3.669325367462664467, 12.12356785135076542, -80.15254291642212081 ) ) ;
#18008=ORIENTED_EDGE ( 'NONE', *, *, #34759, .T. ) ;
#18017=ORIENTED_EDGE ( 'NONE', *, *, #40765, .T. ) ;
#18047=ORIENTED_EDGE ( 'NONE', *, *, #6984, .T. ) ;
#18170=ORIENTED_EDGE ( 'NONE', *, *, #26128, .F. ) ;
#18209=CARTESIAN_POINT ( 'NONE',  ( 0.000000000000000000, 17.49999999999998934, -85.15254291642213502 ) ) ;
#18216=ORIENTED_EDGE ( 'NONE', *, *, #27289, .T. ) ;
#18306=PLANE ( 'NONE',  #676 ) ;
#18403=CARTESIAN_POINT ( 'NONE',  ( 5.376432148649219478, 21.16932536746266535, -85.15254291642213502 ) ) ;
#18428=VERTEX_POINT ( 'NONE', #27130 ) ;
#18458=CARTESIAN_POINT ( 'NONE',  ( 3.876432148649218590, 23.37643214864920438, -80.65254291642212081 ) ) ;
#18472=VECTOR ( 'NONE', #30043, 1000.000000000000000 ) ;
#18495=ADVANCED_FACE ( 'NONE', ( #12426 ), #34975, .T. ) ;
#18509=MECHANICAL_DESIGN_GEOMETRIC_PRESENTATION_REPRESENTATION('',(#11058),#37549);
#18535=CARTESIAN_POINT ( 'NONE',  ( -4.000000000000003553, 17.49999999999998934, -84.65254291642213502 ) ) ;
#18572=ADVANCED_FACE ( 'NONE', ( #15421 ), #9608, .T. ) ;
#18637=ORIENTED_EDGE ( 'NONE', *, *, #12643, .F. ) ;
#18722=ADVANCED_FACE ( 'NONE', ( #39051, #22892 ), #38638, .T. ) ;
#18743=DIRECTION ( 'NONE',  ( 0.000000000000000000, -0.000000000000000000, 1.000000000000000000 ) ) ;
#18881=VERTEX_POINT ( 'NONE', #28589 ) ;
#18921=CARTESIAN_POINT ( 'NONE',  ( -5.876432148649216813, 13.62356785135076365, -84.65254291642213502 ) ) ;
#18991=AXIS2_PLACEMENT_3D ( 'NONE', #31562, #31981, #40717 ) ;
#19023=( BOUNDED_CURVE ( )  B_SPLINE_CURVE ( 3, ( #39193, #32400, #9660, #6869 ),
 .UNSPECIFIED., .F., .F. ) 
 B_SPLINE_CURVE_WITH_KNOTS ( ( 4, 4 ),
 ( 4.712388980384689674, 6.283185307179586232 ),
 .UNSPECIFIED. ) 
 CURVE ( )  GEOMETRIC_REPRESENTATION_ITEM ( )  RATIONAL_B_SPLINE_CURVE ( ( 1.000000000000000000, 0.8047378541243649375, 0.8047378541243649375, 1.000000000000000000 ) ) 
 REPRESENTATION_ITEM ( '' )  );
#19266=ORIENTED_EDGE ( 'NONE', *, *, #20692, .T. ) ;
#19290=DIRECTION ( 'NONE',  ( 0.7071067811865484609, -0.7071067811865467956, 0.000000000000000000 ) ) ;
#19379=VERTEX_POINT ( 'NONE', #12644 ) ;
#19427=CARTESIAN_POINT ( 'NONE',  ( 4.000000000000003553, 17.49999999999998934, -80.15254291642212081 ) ) ;
#19431=CARTESIAN_POINT ( 'NONE',  ( -5.876432148649214149, 21.37643214864921148, -84.94543613523558179 ) ) ;
#19441=( BOUNDED_CURVE ( )  B_SPLINE_CURVE ( 3, ( #18403, #15006, #31373, #2237 ),
 .UNSPECIFIED., .F., .T. ) 
 B_SPLINE_CURVE_WITH_KNOTS ( ( 4, 4 ),
 ( 4.712388980384687898, 6.283185307179586232 ),
 .UNSPECIFIED. ) 
 CURVE ( )  GEOMETRIC_REPRESENTATION_ITEM ( )  RATIONAL_B_SPLINE_CURVE ( ( 1.000000000000000000, 0.8047378541243646044, 0.8047378541243646044, 1.000000000000000000 ) ) 
 REPRESENTATION_ITEM ( '' )  );
#19462=DIRECTION ( 'NONE',  ( 1.000000000000000000, 0.000000000000000000, 0.000000000000000000 ) ) ;
#19524=ORIENTED_EDGE ( 'NONE', *, *, #37071, .T. ) ;
#19607=VERTEX_POINT ( 'NONE', #35553 ) ;
#19644=CIRCLE ( 'NONE', #12853, 4.000000000000003553 ) ;
#19710=CARTESIAN_POINT ( 'NONE',  ( -3.876432148649210152, 11.62356785135076542, -80.65254291642212081 ) ) ;
#19728=CARTESIAN_POINT ( 'NONE',  ( -3.790645711022308628, 11.83067463253731155, -80.15254291642214923 ) ) ;
#19741=CIRCLE ( 'NONE', #13632, 4.000000000000003553 ) ;
#19772=AXIS2_PLACEMENT_3D ( 'NONE', #25620, #22627, #31568 ) ;
#19813=DIRECTION ( 'NONE',  ( -0.000000000000000000, -0.000000000000000000, 1.000000000000000000 ) ) ;
#19834=DIRECTION ( 'NONE',  ( -1.000000000000000000, 0.000000000000000000, 0.000000000000000000 ) ) ;
#19894=CARTESIAN_POINT ( 'NONE',  ( 0.000000000000000000, 17.49999999999998934, -80.65254291642212081 ) ) ;
#19983=LINE ( 'NONE', #16795, #7447 ) ;
#20024=( LENGTH_UNIT ( ) NAMED_UNIT ( * ) SI_UNIT ( .MILLI., .METRE. ) );
#20047=ORIENTED_EDGE ( 'NONE', *, *, #13732, .T. ) ;
#20173=CARTESIAN_POINT ( 'NONE',  ( 5.876432148649220366, 11.62356785135076542, -84.65254291642213502 ) ) ;
#20344=VECTOR ( 'NONE', #2762, 1000.000000000000114 ) ;
#20369=ORIENTED_EDGE ( 'NONE', *, *, #15046, .T. ) ;
#20525=VECTOR ( 'NONE', #16686, 1000.000000000000114 ) ;
#20563=ORIENTED_EDGE ( 'NONE', *, *, #36259, .T. ) ;
#20568=DIRECTION ( 'NONE',  ( 0.000000000000000000, 1.000000000000000000, 0.000000000000000000 ) ) ;
#20593=DIRECTION ( 'NONE',  ( -0.000000000000000000, 0.000000000000000000, -1.000000000000000000 ) ) ;
#20680=EDGE_LOOP ( 'NONE', ( #38509, #19524, #27270, #29073 ) ) ;
#20692=EDGE_CURVE ( 'NONE', #11015, #10530, #9300, .T. ) ;
#20805=LINE ( 'NONE', #39940, #4721 ) ;
#20839=CARTESIAN_POINT ( 'NONE',  ( -5.876432148649216813, 13.62356785135076365, -85.15254291642213502 ) ) ;
#20878=CYLINDRICAL_SURFACE ( 'NONE', #33576, 0.5000000000000004441 ) ;
#20888=EDGE_LOOP ( 'NONE', ( #5674, #10208, #37570, #18170 ) ) ;
#20938=ORIENTED_EDGE ( 'NONE', *, *, #11065, .T. ) ;
#20943=DIRECTION ( 'NONE',  ( 1.000000000000000000, 0.000000000000000000, 0.000000000000000000 ) ) ;
#21033=DIRECTION ( 'NONE',  ( 0.000000000000000000, 0.000000000000000000, 1.000000000000000000 ) ) ;
#21094=ORIENTED_EDGE ( 'NONE', *, *, #38353, .T. ) ;
#21101=EDGE_CURVE ( 'NONE', #21607, #32392, #36731, .T. ) ;
#21180=ORIENTED_EDGE ( 'NONE', *, *, #28386, .F. ) ;
#21201=ORIENTED_EDGE ( 'NONE', *, *, #35585, .F. ) ;
#21205=DIRECTION ( 'NONE',  ( 0.000000000000000000, 0.000000000000000000, 1.000000000000000000 ) ) ;
#21264=EDGE_CURVE ( 'NONE', #41881, #37165, #34787, .T. ) ;
#21275=AXIS2_PLACEMENT_3D ( 'NONE', #18535, #4930, #40869 ) ;
#21315=EDGE_CURVE ( 'NONE', #38251, #40492, #14411, .T. ) ;
#21393=FACE_OUTER_BOUND ( 'NONE', #4940, .T. ) ;
#21410=DIRECTION ( 'NONE',  ( -0.000000000000000000, -1.000000000000000000, -0.000000000000000000 ) ) ;
#21565=ORIENTED_EDGE ( 'NONE', *, *, #14813, .F. ) ;
#21607=VERTEX_POINT ( 'NONE', #30467 ) ;
#21627=EDGE_LOOP ( 'NONE', ( #26074, #2474, #30352, #29940, #36255, #34207, #22876, #2561 ) ) ;
#21674=AXIS2_PLACEMENT_3D ( 'NONE', #31885, #25732, #32101 ) ;
#21676=EDGE_CURVE ( 'NONE', #24594, #15673, #14101, .T. ) ;
#21718=DIRECTION ( 'NONE',  ( -0.7071067811865484609, 0.7071067811865465735, 0.000000000000000000 ) ) ;
#21723=LINE ( 'NONE', #11317, #33711 ) ;
#21730=VERTEX_POINT ( 'NONE', #33020 ) ;
#21754=( BOUNDED_CURVE ( )  B_SPLINE_CURVE ( 3, ( #27417, #11247, #30809, #24023 ),
 .UNSPECIFIED., .F., .T. ) 
 B_SPLINE_CURVE_WITH_KNOTS ( ( 4, 4 ),
 ( 4.712388980384691450, 6.283185307179586232 ),
 .UNSPECIFIED. ) 
 CURVE ( )  GEOMETRIC_REPRESENTATION_ITEM ( )  RATIONAL_B_SPLINE_CURVE ( ( 1.000000000000000000, 0.8047378541243654926, 0.8047378541243654926, 1.000000000000000000 ) ) 
 REPRESENTATION_ITEM ( '' )  );
#21811=( BOUNDED_CURVE ( )  B_SPLINE_CURVE ( 3, ( #8876, #41852, #38643, #2917 ),
 .UNSPECIFIED., .F., .F. ) 
 B_SPLINE_CURVE_WITH_KNOTS ( ( 4, 4 ),
 ( 0.000000000000000000, 1.570796326794899889 ),
 .UNSPECIFIED. ) 
 CURVE ( )  GEOMETRIC_REPRESENTATION_ITEM ( )  RATIONAL_B_SPLINE_CURVE ( ( 1.000000000000000000, 0.8047378541243641603, 0.8047378541243641603, 1.000000000000000000 ) ) 
 REPRESENTATION_ITEM ( '' )  );
#21872=CYLINDRICAL_SURFACE ( 'NONE', #4249, 0.5000000000000004441 ) ;
#21933=VECTOR ( 'NONE', #15688, 1000.000000000000114 ) ;
#22062=LINE ( 'NONE', #25681, #30102 ) ;
#22097=( GEOMETRIC_REPRESENTATION_CONTEXT ( 3 ) GLOBAL_UNCERTAINTY_ASSIGNED_CONTEXT ( ( #5892 ) ) GLOBAL_UNIT_ASSIGNED_CONTEXT ( ( #1552, #31306, #28114 ) ) REPRESENTATION_CONTEXT ( 'NONE', 'WORKASPACE' ) );
#22176=CARTESIAN_POINT ( 'NONE',  ( -5.876432148649216813, 21.37643214864921504, -80.35964969760868826 ) ) ;
#22194=EDGE_CURVE ( 'NONE', #19607, #34859, #20805, .T. ) ;
#22211=EDGE_CURVE ( 'NONE', #15190, #40461, #19644, .T. ) ;
#22231=CARTESIAN_POINT ( 'NONE',  ( 13.27287875805592776, 13.27287875805599704, -80.65254291642212081 ) ) ;
#22240=ORIENTED_EDGE ( 'NONE', *, *, #34782, .T. ) ;
#22246=CARTESIAN_POINT ( 'NONE',  ( -5.376432148649216813, 13.62356785135076365, -80.15254291642212081 ) ) ;
#22264=DIRECTION ( 'NONE',  ( 1.000000000000000000, -0.000000000000000000, -0.000000000000000000 ) ) ;
#22294=CARTESIAN_POINT ( 'NONE',  ( -5.376432148649216813, 0.000000000000000000, -84.65254291642213502 ) ) ;
#22355=ORIENTED_EDGE ( 'NONE', *, *, #36318, .F. ) ;
#22366=AXIS2_PLACEMENT_3D ( 'NONE', #9994, #15747, #35924 ) ;
#22627=DIRECTION ( 'NONE',  ( 0.000000000000000000, -0.000000000000000000, 1.000000000000000000 ) ) ;
#22709=LINE ( 'NONE', #28451, #5580 ) ;
#22753=CARTESIAN_POINT ( 'NONE',  ( 5.876432148649220366, 12.12356785135076542, -80.65254291642212081 ) ) ;
#22807=DIRECTION ( 'NONE',  ( 1.000000000000000000, -0.000000000000000000, 0.000000000000000000 ) ) ;
#22814=VECTOR ( 'NONE', #38710, 1000.000000000000000 ) ;
#22860=DIRECTION ( 'NONE',  ( 0.000000000000000000, 0.000000000000000000, -1.000000000000000000 ) ) ;
#22870=ORIENTED_EDGE ( 'NONE', *, *, #40765, .F. ) ;
#22876=ORIENTED_EDGE ( 'NONE', *, *, #21264, .T. ) ;
#22892=FACE_OUTER_BOUND ( 'NONE', #21627, .T. ) ;
#22932=( BOUNDED_CURVE ( )  B_SPLINE_CURVE ( 3, ( #9414, #22176, #32166, #38130 ),
 .UNSPECIFIED., .F., .F. ) 
 B_SPLINE_CURVE_WITH_KNOTS ( ( 4, 4 ),
 ( 3.141592653589793116, 4.712388980384689674 ),
 .UNSPECIFIED. ) 
 CURVE ( )  GEOMETRIC_REPRESENTATION_ITEM ( )  RATIONAL_B_SPLINE_CURVE ( ( 1.000000000000000000, 0.8047378541243649375, 0.8047378541243649375, 1.000000000000000000 ) ) 
 REPRESENTATION_ITEM ( '' )  );
#22956=FACE_OUTER_BOUND ( 'NONE', #23077, .T. ) ;
#22999=EDGE_CURVE ( 'NONE', #24919, #40492, #37330, .T. ) ;
#23038=EDGE_CURVE ( 'NONE', #11015, #32392, #33437, .T. ) ;
#23056=EDGE_CURVE ( 'NONE', #5251, #16965, #19023, .T. ) ;
#23077=EDGE_LOOP ( 'NONE', ( #8641, #2601, #24452, #12388 ) ) ;
#23151=CARTESIAN_POINT ( 'NONE',  ( 5.876432148649220366, 13.62356785135077075, -84.65254291642213502 ) ) ;
#23182=ORIENTED_EDGE ( 'NONE', *, *, #2845, .F. ) ;
#23279=AXIS2_PLACEMENT_3D ( 'NONE', #32445, #747, #29451 ) ;
#23370=DIRECTION ( 'NONE',  ( -0.7071067811865493491, 0.7071067811865456854, -0.000000000000000000 ) ) ;
#23450=ORIENTED_EDGE ( 'NONE', *, *, #27437, .F. ) ;
#23535=DIRECTION ( 'NONE',  ( 1.224646799147353207E-16, 1.000000000000000000, 0.000000000000000000 ) ) ;
#23636=EDGE_CURVE ( 'NONE', #8374, #24919, #24457, .T. ) ;
#23680=EDGE_CURVE ( 'NONE', #14391, #39500, #21754, .T. ) ;
#23711=DIRECTION ( 'NONE',  ( -1.000000000000000000, 0.000000000000000000, 0.000000000000000000 ) ) ;
#23818=DIRECTION ( 'NONE',  ( -0.7071067811865469066, -0.7071067811865482389, -0.000000000000000000 ) ) ;
#23827=LINE ( 'NONE', #20839, #16287 ) ;
#23873=DIRECTION ( 'NONE',  ( 0.000000000000000000, 0.000000000000000000, -1.000000000000000000 ) ) ;
#23939=CARTESIAN_POINT ( 'NONE',  ( 0.000000000000000000, 17.49999999999998934, -85.15254291642213502 ) ) ;
#24004=VECTOR ( 'NONE', #10646, 999.9999999999998863 ) ;
#24023=CARTESIAN_POINT ( 'NONE',  ( -3.876432148649222142, 23.37643214864920438, -84.65254291642213502 ) ) ;
#24031=DIRECTION ( 'NONE',  ( 0.7071067811865465735, 0.7071067811865483499, -0.000000000000000000 ) ) ;
#24041=CIRCLE ( 'NONE', #9766, 3.500000000000003997 ) ;
#24084=FACE_OUTER_BOUND ( 'NONE', #33214, .T. ) ;
#24111=AXIS2_PLACEMENT_3D ( 'NONE', #3745, #13117, #19290 ) ;
#24112=DIRECTION ( 'NONE',  ( 0.000000000000000000, 0.000000000000000000, 1.000000000000000000 ) ) ;
#24263=ADVANCED_FACE ( 'NONE', ( #9152 ), #18306, .F. ) ;
#24452=ORIENTED_EDGE ( 'NONE', *, *, #22999, .T. ) ;
#24457=CIRCLE ( 'NONE', #28512, 3.500000000000003997 ) ;
#24461=EDGE_CURVE ( 'NONE', #10530, #19379, #23827, .T. ) ;
#24496=EDGE_LOOP ( 'NONE', ( #39084, #12887, #20563, #10961 ) ) ;
#24509=DIRECTION ( 'NONE',  ( 1.000000000000000000, 0.000000000000000000, 0.000000000000000000 ) ) ;
#24532=DIRECTION ( 'NONE',  ( -0.7071067811865459074, -0.7071067811865493491, 0.000000000000000000 ) ) ;
#24589=LINE ( 'NONE', #37970, #2058 ) ;
#24594=VERTEX_POINT ( 'NONE', #30404 ) ;
#24604=ORIENTED_EDGE ( 'NONE', *, *, #36963, .F. ) ;
#24620=DIRECTION ( 'NONE',  ( 0.000000000000000000, 0.000000000000000000, -1.000000000000000000 ) ) ;
#24641=CARTESIAN_POINT ( 'NONE',  ( 5.876432148649220366, 13.62356785135077075, -80.65254291642212081 ) ) ;
#24659=ORIENTED_EDGE ( 'NONE', *, *, #7673, .T. ) ;
#24661=EDGE_CURVE ( 'NONE', #41881, #37786, #12811, .T. ) ;
#24752=( BOUNDED_CURVE ( )  B_SPLINE_CURVE ( 3, ( #36304, #3765, #16749, #7380 ),
 .UNSPECIFIED., .F., .T. ) 
 B_SPLINE_CURVE_WITH_KNOTS ( ( 4, 4 ),
 ( 0.000000000000000000, 1.570796326794896558 ),
 .UNSPECIFIED. ) 
 CURVE ( )  GEOMETRIC_REPRESENTATION_ITEM ( )  RATIONAL_B_SPLINE_CURVE ( ( 1.000000000000000000, 0.8047378541243649375, 0.8047378541243649375, 1.000000000000000000 ) ) 
 REPRESENTATION_ITEM ( '' )  );
#24813=DIRECTION ( 'NONE',  ( -0.000000000000000000, 1.000000000000000000, -0.000000000000000000 ) ) ;
#24845=VECTOR ( 'NONE', #34412, 1000.000000000000000 ) ;
#24862=DIRECTION ( 'NONE',  ( 0.000000000000000000, 0.000000000000000000, 1.000000000000000000 ) ) ;
#24874=AXIS2_PLACEMENT_3D ( 'NONE', #4632, #40365, #8033 ) ;
#24896=EDGE_CURVE ( 'NONE', #34859, #4624, #7092, .T. ) ;
#24919=VERTEX_POINT ( 'NONE', #25278 ) ;
#25056=CARTESIAN_POINT ( 'NONE',  ( -5.376432148649216813, 13.83067463253730978, -80.15254291642212081 ) ) ;
#25134=ORIENTED_EDGE ( 'NONE', *, *, #24661, .F. ) ;
#25157=AXIS2_PLACEMENT_3D ( 'NONE', #31705, #21718, #18743 ) ;
#25173=EDGE_CURVE ( 'NONE', #34634, #4624, #32525, .T. ) ;
#25187=ADVANCED_FACE ( 'NONE', ( #22956 ), #40708, .T. ) ;
#25250=ORIENTED_EDGE ( 'NONE', *, *, #21315, .T. ) ;
#25278=CARTESIAN_POINT ( 'NONE',  ( 3.500000000000003997, 17.49999999999998934, -84.65254291642213502 ) ) ;
#25282=EDGE_CURVE ( 'NONE', #39500, #11015, #36354, .T. ) ;
#25285=ORIENTED_EDGE ( 'NONE', *, *, #7409, .F. ) ;
#25288=AXIS2_PLACEMENT_3D ( 'NONE', #3816, #13595, #24862 ) ;
#25296=EDGE_LOOP ( 'NONE', ( #25711, #11612, #36685, #6404 ) ) ;
#25343=EDGE_CURVE ( 'NONE', #21730, #41881, #19983, .T. ) ;
#25620=CARTESIAN_POINT ( 'NONE',  ( 0.000000000000000000, 17.49999999999998934, -80.65254291642212081 ) ) ;
#25681=CARTESIAN_POINT ( 'NONE',  ( 3.876432148649220366, 12.12356785135076542, -80.15254291642212081 ) ) ;
#25686=DIRECTION ( 'NONE',  ( 0.7071067811865460184, 0.7071067811865491270, 0.000000000000000000 ) ) ;
#25708=ADVANCED_FACE ( 'NONE', ( #28450 ), #35687, .T. ) ;
#25711=ORIENTED_EDGE ( 'NONE', *, *, #36060, .T. ) ;
#25732=DIRECTION ( 'NONE',  ( 0.000000000000000000, 1.000000000000000000, 0.000000000000000000 ) ) ;
#25745=LINE ( 'NONE', #5753, #22814 ) ;
#25817=CARTESIAN_POINT ( 'NONE',  ( 0.000000000000000000, 12.12356785135076542, -84.65254291642213502 ) ) ;
#25867=FACE_OUTER_BOUND ( 'NONE', #147, .T. ) ;
#25900=ORIENTED_EDGE ( 'NONE', *, *, #36966, .T. ) ;
#25919=CARTESIAN_POINT ( 'NONE',  ( -3.876432148649229248, 23.37643214864920438, -80.35964969760867405 ) ) ;
#25936=EDGE_CURVE ( 'NONE', #19379, #34634, #24752, .T. ) ;
#26008=CARTESIAN_POINT ( 'NONE',  ( -5.876432148649216813, 11.62356785135076542, -85.15254291642213502 ) ) ;
#26074=ORIENTED_EDGE ( 'NONE', *, *, #21676, .T. ) ;
#26079=AXIS2_PLACEMENT_3D ( 'NONE', #26008, #22807, #35779 ) ;
#26128=EDGE_CURVE ( 'NONE', #5251, #17850, #27725, .T. ) ;
#26132=CARTESIAN_POINT ( 'NONE',  ( -3.790645711022324171, 23.16932536746265825, -80.15254291642212081 ) ) ;
#26187=VERTEX_POINT ( 'NONE', #28140 ) ;
#26203=CYLINDRICAL_SURFACE ( 'NONE', #3569, 0.5000000000000004441 ) ;
#26216=FACE_OUTER_BOUND ( 'NONE', #11825, .T. ) ;
#26444=VECTOR ( 'NONE', #23818, 999.9999999999998863 ) ;
#26465=DIRECTION ( 'NONE',  ( 0.000000000000000000, 0.000000000000000000, -1.000000000000000000 ) ) ;
#26609=ADVANCED_FACE ( 'NONE', ( #2499 ), #8665, .F. ) ;
#26610=CARTESIAN_POINT ( 'NONE',  ( 5.876432148649220366, 21.37643214864921148, -84.65254291642213502 ) ) ;
#26679=ORIENTED_EDGE ( 'NONE', *, *, #23038, .T. ) ;
#26754=AXIS2_PLACEMENT_3D ( 'NONE', #6841, #19813, #460 ) ;
#26780=CARTESIAN_POINT ( 'NONE',  ( 5.876432148649220366, 23.37643214864920438, -85.15254291642213502 ) ) ;
#26892=ORIENTED_EDGE ( 'NONE', *, *, #37071, .F. ) ;
#26955=CARTESIAN_POINT ( 'NONE',  ( 5.376432148649220366, 0.000000000000000000, -84.65254291642213502 ) ) ;
#26969=EDGE_LOOP ( 'NONE', ( #13357, #16000, #1996, #16603 ) ) ;
#27037=DIRECTION ( 'NONE',  ( 0.7071067811865482389, -0.7071067811865469066, 0.000000000000000000 ) ) ;
#27074=CARTESIAN_POINT ( 'NONE',  ( -3.876432148649222142, 22.87643214864920438, -80.15254291642212081 ) ) ;
#27118=FACE_OUTER_BOUND ( 'NONE', #15032, .T. ) ;
#27130=CARTESIAN_POINT ( 'NONE',  ( -3.876432148649210152, 11.62356785135076542, -84.65254291642213502 ) ) ;
#27208=DIRECTION ( 'NONE',  ( -0.000000000000000000, 0.000000000000000000, -1.000000000000000000 ) ) ;
#27262=DIRECTION ( 'NONE',  ( 0.7071067811865484609, -0.7071067811865467956, 0.000000000000000000 ) ) ;
#27270=ORIENTED_EDGE ( 'NONE', *, *, #36060, .F. ) ;
#27278=VERTEX_POINT ( 'NONE', #31376 ) ;
#27289=EDGE_CURVE ( 'NONE', #10530, #18428, #24589, .T. ) ;
#27314=DIRECTION ( 'NONE',  ( 1.000000000000000000, 0.000000000000000000, 0.000000000000000000 ) ) ;
#27316=ORIENTED_EDGE ( 'NONE', *, *, #11065, .F. ) ;
#27317=VECTOR ( 'NONE', #24813, 1000.000000000000000 ) ;
#27417=CARTESIAN_POINT ( 'NONE',  ( -3.669325367462682230, 22.87643214864920438, -85.15254291642213502 ) ) ;
#27437=EDGE_CURVE ( 'NONE', #37991, #16965, #13069, .T. ) ;
#27484=EDGE_LOOP ( 'NONE', ( #29771, #40258, #37465, #36531 ) ) ;
#27525=ORIENTED_EDGE ( 'NONE', *, *, #27289, .F. ) ;
#27532=CARTESIAN_POINT ( 'NONE',  ( -5.876432148649216813, 21.37643214864920438, -80.65254291642212081 ) ) ;
#27721=EDGE_CURVE ( 'NONE', #40492, #38251, #29216, .T. ) ;
#27725=LINE ( 'NONE', #41546, #34640 ) ;
#27856=CARTESIAN_POINT ( 'NONE',  ( 3.876432148649223475, 11.62356785135076898, -84.94543613523559600 ) ) ;
#27895=CARTESIAN_POINT ( 'NONE',  ( -4.000000000000003553, 17.49999999999998934, -80.15254291642212081 ) ) ;
#27940=AXIS2_PLACEMENT_3D ( 'NONE', #12638, #6042, #28585 ) ;
#28114=( NAMED_UNIT ( * ) SI_UNIT ( $, .STERADIAN. ) SOLID_ANGLE_UNIT ( ) );
#28140=CARTESIAN_POINT ( 'NONE',  ( 5.876432148649220366, 21.37643214864921148, -80.65254291642212081 ) ) ;
#28224=PRODUCT ( 'Square Nut', 'Square Nut', '', ( #13724 ) ) ;
#28260=CIRCLE ( 'NONE', #9937, 0.5000000000000004441 ) ;
#28310=CARTESIAN_POINT ( 'NONE',  ( 0.000000000000000000, 22.87643214864920438, -85.15254291642213502 ) ) ;
#28386=EDGE_CURVE ( 'NONE', #17850, #5925, #37456, .T. ) ;
#28416=CARTESIAN_POINT ( 'NONE',  ( 5.376432148649220366, 21.16932536746266180, -80.15254291642212081 ) ) ;
#28450=FACE_OUTER_BOUND ( 'NONE', #29931, .T. ) ;
#28451=CARTESIAN_POINT ( 'NONE',  ( 5.876432148649220366, 23.37643214864920438, -84.65254291642213502 ) ) ;
#28509=ORIENTED_EDGE ( 'NONE', *, *, #26128, .T. ) ;
#28512=AXIS2_PLACEMENT_3D ( 'NONE', #1873, #27208, #14854 ) ;
#28585=DIRECTION ( 'NONE',  ( 0.7071067811865457964, 0.7071067811865492381, 0.000000000000000000 ) ) ;
#28589=CARTESIAN_POINT ( 'NONE',  ( 3.500000000000003997, 17.49999999999998934, -80.65254291642212081 ) ) ;
#28706=ORIENTED_EDGE ( 'NONE', *, *, #21101, .T. ) ;
#28891=PRODUCT_DEFINITION_FORMATION_WITH_SPECIFIED_SOURCE ( 'ANY', '', #28224, .NOT_KNOWN. ) ;
#28916=FACE_OUTER_BOUND ( 'NONE', #26969, .T. ) ;
#28948=ADVANCED_FACE ( 'NONE', ( #21393 ), #1215, .T. ) ;
#29044=ADVANCED_FACE ( 'NONE', ( #2249 ), #9049, .T. ) ;
#29073=ORIENTED_EDGE ( 'NONE', *, *, #11318, .T. ) ;
#29093=PRODUCT_DEFINITION ( 'UNKNOWN', '', #28891, #6722 ) ;
#29170=PLANE ( 'NONE',  #26079 ) ;
#29216=CIRCLE ( 'NONE', #10905, 4.000000000000003553 ) ;
#29246=VECTOR ( 'NONE', #5325, 1000.000000000000000 ) ;
#29310=DIRECTION ( 'NONE',  ( 0.000000000000000000, 0.000000000000000000, -1.000000000000000000 ) ) ;
#29391=ORIENTED_EDGE ( 'NONE', *, *, #28386, .T. ) ;
#29451=DIRECTION ( 'NONE',  ( 1.000000000000000000, 0.000000000000000000, -0.000000000000000000 ) ) ;
#29476=DIRECTION ( 'NONE',  ( -0.000000000000000000, -1.000000000000000000, -0.000000000000000000 ) ) ;
#29547=FACE_OUTER_BOUND ( 'NONE', #3931, .T. ) ;
#29675=CARTESIAN_POINT ( 'NONE',  ( -3.876432148649222142, 23.37643214864920438, -80.65254291642212081 ) ) ;
#29771=ORIENTED_EDGE ( 'NONE', *, *, #514, .F. ) ;
#29827=CARTESIAN_POINT ( 'NONE',  ( -3.876432148649215481, 11.62356785135076720, -84.94543613523558179 ) ) ;
#29832=CARTESIAN_POINT ( 'NONE',  ( -5.876432148649217702, 13.62356785135076187, -84.94543613523558179 ) ) ;
#29931=EDGE_LOOP ( 'NONE', ( #13301, #15131, #2983, #24604 ) ) ;
#29940=ORIENTED_EDGE ( 'NONE', *, *, #25173, .T. ) ;
#29950=CARTESIAN_POINT ( 'NONE',  ( 5.876432148649220366, 21.37643214864921148, -80.65254291642212081 ) ) ;
#30043=DIRECTION ( 'NONE',  ( -1.000000000000000000, -0.000000000000000000, 0.000000000000000000 ) ) ;
#30076=CARTESIAN_POINT ( 'NONE',  ( 5.876432148649220366, 11.62356785135076542, -85.15254291642213502 ) ) ;
#30102=VECTOR ( 'NONE', #22264, 1000.000000000000000 ) ;
#30275=CARTESIAN_POINT ( 'NONE',  ( 0.000000000000000000, 17.49999999999998934, -84.65254291642213502 ) ) ;
#30352=ORIENTED_EDGE ( 'NONE', *, *, #37101, .T. ) ;
#30404=CARTESIAN_POINT ( 'NONE',  ( 3.669325367462669796, 22.87643214864920438, -80.15254291642212081 ) ) ;
#30467=CARTESIAN_POINT ( 'NONE',  ( -5.376432148649216813, 13.83067463253730978, -85.15254291642213502 ) ) ;
#30570=LINE ( 'NONE', #36746, #9659 ) ;
#30809=CARTESIAN_POINT ( 'NONE',  ( -3.876432148649226583, 23.37643214864920438, -84.94543613523558179 ) ) ;
#30853=PLANE ( 'NONE',  #21674 ) ;
#30942=CARTESIAN_POINT ( 'NONE',  ( 0.000000000000000000, 17.49999999999998934, -80.15254291642212081 ) ) ;
#30989=EDGE_LOOP ( 'NONE', ( #21094, #35524, #7127, #9953 ) ) ;
#31077=CARTESIAN_POINT ( 'NONE',  ( 5.876432148649220366, 21.37643214864921148, -85.15254291642213502 ) ) ;
#31091=ORIENTED_EDGE ( 'NONE', *, *, #36966, .F. ) ;
#31120=CARTESIAN_POINT ( 'NONE',  ( -5.376432148649216813, 21.16932536746266535, -80.15254291642212081 ) ) ;
#31196=DIRECTION ( 'NONE',  ( 1.000000000000000000, -0.000000000000000000, -0.000000000000000000 ) ) ;
#31231=CARTESIAN_POINT ( 'NONE',  ( 5.669325367462673348, 13.70935428897767316, -80.15254291642210660 ) ) ;
#31237=EDGE_LOOP ( 'NONE', ( #3161, #18637, #7768, #31553 ) ) ;
#31306=( NAMED_UNIT ( * ) PLANE_ANGLE_UNIT ( ) SI_UNIT ( $, .RADIAN. ) );
#31373=CARTESIAN_POINT ( 'NONE',  ( 5.876432148649222142, 21.37643214864921504, -84.94543613523558179 ) ) ;
#31376=CARTESIAN_POINT ( 'NONE',  ( 3.876432148649220366, 11.62356785135076542, -84.65254291642213502 ) ) ;
#31400=LINE ( 'NONE', #2266, #14041 ) ;
#31402=CARTESIAN_POINT ( 'NONE',  ( 3.876432148649218590, 23.37643214864920438, -84.65254291642213502 ) ) ;
#31405=DIRECTION ( 'NONE',  ( 0.000000000000000000, -1.000000000000000000, -0.000000000000000000 ) ) ;
#31553=ORIENTED_EDGE ( 'NONE', *, *, #15046, .F. ) ;
#31561=LINE ( 'NONE', #11573, #343 ) ;
#31562=CARTESIAN_POINT ( 'NONE',  ( 4.000000000000003553, 17.49999999999998934, -84.65254291642213502 ) ) ;
#31568=DIRECTION ( 'NONE',  ( 1.000000000000000000, 0.000000000000000000, 0.000000000000000000 ) ) ;
#31636=ORIENTED_EDGE ( 'NONE', *, *, #23636, .F. ) ;
#31654=FACE_OUTER_BOUND ( 'NONE', #36458, .T. ) ;
#31705=CARTESIAN_POINT ( 'NONE',  ( 3.876432148649220366, 11.62356785135076542, -85.15254291642213502 ) ) ;
#31807=ORIENTED_EDGE ( 'NONE', *, *, #36798, .F. ) ;
#31885=CARTESIAN_POINT ( 'NONE',  ( 5.876432148649220366, 11.62356785135076542, -85.15254291642213502 ) ) ;
#31894=CARTESIAN_POINT ( 'NONE',  ( 4.227121241944059804, 4.227121241944077568, -80.15254291642212081 ) ) ;
#31939=CARTESIAN_POINT ( 'NONE',  ( -5.376432148649216813, 11.62356785135076542, -80.65254291642212081 ) ) ;
#31955=ORIENTED_EDGE ( 'NONE', *, *, #9497, .F. ) ;
#31981=DIRECTION ( 'NONE',  ( 0.000000000000000000, -1.000000000000000000, -0.000000000000000000 ) ) ;
#32079=DIRECTION ( 'NONE',  ( -0.7071067811865490160, 0.7071067811865460184, 0.000000000000000000 ) ) ;
#32101=DIRECTION ( 'NONE',  ( 0.000000000000000000, -0.000000000000000000, 1.000000000000000000 ) ) ;
#32112=CYLINDRICAL_SURFACE ( 'NONE', #34179, 0.5000000000000004441 ) ;
#32155=CARTESIAN_POINT ( 'NONE',  ( 5.376432148649220366, 13.83067463253731688, -85.15254291642213502 ) ) ;
#32166=CARTESIAN_POINT ( 'NONE',  ( -5.669325367462668908, 21.29064571102230730, -80.15254291642210660 ) ) ;
#32283=FACE_OUTER_BOUND ( 'NONE', #41864, .T. ) ;
#32290=ORIENTED_EDGE ( 'NONE', *, *, #24461, .T. ) ;
#32304=CARTESIAN_POINT ( 'NONE',  ( 3.876432148649218590, 23.37643214864920438, -84.65254291642213502 ) ) ;
#32392=VERTEX_POINT ( 'NONE', #16161 ) ;
#32400=CARTESIAN_POINT ( 'NONE',  ( 3.790645711022312181, 23.16932536746264759, -85.15254291642212081 ) ) ;
#32404=EDGE_CURVE ( 'NONE', #3668, #16965, #35710, .T. ) ;
#32445=CARTESIAN_POINT ( 'NONE',  ( 0.000000000000000000, 0.000000000000000000, -85.15254291642213502 ) ) ;
#32448=FACE_OUTER_BOUND ( 'NONE', #16613, .T. ) ;
#32468=FACE_OUTER_BOUND ( 'NONE', #39137, .T. ) ;
#32470=EDGE_CURVE ( 'NONE', #37165, #24594, #39301, .T. ) ;
#32525=LINE ( 'NONE', #31894, #20344 ) ;
#32595=DIRECTION ( 'NONE',  ( 0.000000000000000000, 0.000000000000000000, 1.000000000000000000 ) ) ;
#32600=EDGE_CURVE ( 'NONE', #37165, #26187, #1995, .T. ) ;
#32697=CARTESIAN_POINT ( 'NONE',  ( -3.669325367462664467, 12.12356785135076542, -80.15254291642212081 ) ) ;
#32725=( BOUNDED_CURVE ( )  B_SPLINE_CURVE ( 3, ( #13355, #26132, #25919, #39086 ),
 .UNSPECIFIED., .F., .T. ) 
 B_SPLINE_CURVE_WITH_KNOTS ( ( 4, 4 ),
 ( 4.712388980384688786, 6.283185307179586232 ),
 .UNSPECIFIED. ) 
 CURVE ( )  GEOMETRIC_REPRESENTATION_ITEM ( )  RATIONAL_B_SPLINE_CURVE ( ( 1.000000000000000000, 0.8047378541243648264, 0.8047378541243648264, 1.000000000000000000 ) ) 
 REPRESENTATION_ITEM ( '' )  );
#32956=DIRECTION ( 'NONE',  ( 0.000000000000000000, 0.000000000000000000, 1.000000000000000000 ) ) ;
#32999=CYLINDRICAL_SURFACE ( 'NONE', #26754, 3.500000000000003997 ) ;
#33020=CARTESIAN_POINT ( 'NONE',  ( 3.669325367462673793, 12.12356785135076542, -80.15254291642212081 ) ) ;
#33166=ORIENTED_EDGE ( 'NONE', *, *, #5823, .F. ) ;
#33214=EDGE_LOOP ( 'NONE', ( #22240, #8279, #31955, #209 ) ) ;
#33278=DIRECTION ( 'NONE',  ( -0.000000000000000000, -0.000000000000000000, 1.000000000000000000 ) ) ;
#33380=AXIS2_PLACEMENT_3D ( 'NONE', #35858, #6933, #3527 ) ;
#33437=( BOUNDED_CURVE ( )  B_SPLINE_CURVE ( 3, ( #13049, #19431, #16052, #6461 ),
 .UNSPECIFIED., .F., .T. ) 
 B_SPLINE_CURVE_WITH_KNOTS ( ( 4, 4 ),
 ( 0.000000000000000000, 1.570796326794895226 ),
 .UNSPECIFIED. ) 
 CURVE ( )  GEOMETRIC_REPRESENTATION_ITEM ( )  RATIONAL_B_SPLINE_CURVE ( ( 1.000000000000000000, 0.8047378541243652705, 0.8047378541243652705, 1.000000000000000000 ) ) 
 REPRESENTATION_ITEM ( '' )  );
#33467=FACE_OUTER_BOUND ( 'NONE', #5979, .T. ) ;
#33547=CARTESIAN_POINT ( 'NONE',  ( 3.500000000000003997, 17.49999999999998934, -85.15254291642213502 ) ) ;
#33576=AXIS2_PLACEMENT_3D ( 'NONE', #40640, #33849, #14501 ) ;
#33578=CARTESIAN_POINT ( 'NONE',  ( 5.876432148649220366, 21.37643214864921504, -80.35964969760865984 ) ) ;
#33638=AXIS2_PLACEMENT_3D ( 'NONE', #14064, #27037, #10446 ) ;
#33650=CARTESIAN_POINT ( 'NONE',  ( 3.876432148649218590, 23.37643214864920438, -80.65254291642212081 ) ) ;
#33667=ORIENTED_EDGE ( 'NONE', *, *, #27721, .T. ) ;
#33711=VECTOR ( 'NONE', #37273, 1000.000000000000000 ) ;
#33777=FACE_OUTER_BOUND ( 'NONE', #13930, .T. ) ;
#33849=DIRECTION ( 'NONE',  ( -1.000000000000000000, 0.000000000000000000, 0.000000000000000000 ) ) ;
#33874=ORIENTED_EDGE ( 'NONE', *, *, #1147, .F. ) ;
#33912=ADVANCED_FACE ( 'NONE', ( #33467 ), #2397, .T. ) ;
#34043=FACE_OUTER_BOUND ( 'NONE', #25296, .T. ) ;
#34179=AXIS2_PLACEMENT_3D ( 'NONE', #22753, #16384, #38280 ) ;
#34207=ORIENTED_EDGE ( 'NONE', *, *, #25343, .T. ) ;
#34229=APPLICATION_CONTEXT ( 'automotive_design' ) ;
#34237=AXIS2_PLACEMENT_3D ( 'NONE', #39647, #19462, #22860 ) ;
#34338=DIRECTION ( 'NONE',  ( -0.000000000000000000, 0.000000000000000000, -1.000000000000000000 ) ) ;
#34394=VECTOR ( 'NONE', #1027, 999.9999999999998863 ) ;
#34412=DIRECTION ( 'NONE',  ( 0.000000000000000000, -1.000000000000000000, 0.000000000000000000 ) ) ;
#34483=PLANE ( 'NONE',  #25157 ) ;
#34617=CARTESIAN_POINT ( 'NONE',  ( 3.790645711022314401, 23.16932536746264759, -80.15254291642210660 ) ) ;
#34634=VERTEX_POINT ( 'NONE', #25056 ) ;
#34640=VECTOR ( 'NONE', #9209, 1000.000000000000000 ) ;
#34759=EDGE_CURVE ( 'NONE', #26187, #37786, #14850, .T. ) ;
#34782=EDGE_CURVE ( 'NONE', #24594, #37991, #7279, .T. ) ;
#34787=LINE ( 'NONE', #4816, #27317 ) ;
#34836=LINE ( 'NONE', #9314, #11078 ) ;
#34846=VECTOR ( 'NONE', #8889, 1000.000000000000000 ) ;
#34859=VERTEX_POINT ( 'NONE', #19710 ) ;
#34925=CARTESIAN_POINT ( 'NONE',  ( 5.876432148649222142, 13.62356785135076898, -84.94543613523558179 ) ) ;
#34975=CYLINDRICAL_SURFACE ( 'NONE', #27940, 0.4999999999999994449 ) ;
#35126=SHAPE_REPRESENTATION_RELATIONSHIP ( 'NONE' , 'NONE' ,  #10382, #40622 ) ;
#35218=( BOUNDED_CURVE ( )  B_SPLINE_CURVE ( 3, ( #4727, #29827, #13881, #40036 ),
 .UNSPECIFIED., .F., .T. ) 
 B_SPLINE_CURVE_WITH_KNOTS ( ( 4, 4 ),
 ( 0.000000000000000000, 1.570796326794896558 ),
 .UNSPECIFIED. ) 
 CURVE ( )  GEOMETRIC_REPRESENTATION_ITEM ( )  RATIONAL_B_SPLINE_CURVE ( ( 1.000000000000000000, 0.8047378541243649375, 0.8047378541243649375, 1.000000000000000000 ) ) 
 REPRESENTATION_ITEM ( '' )  );
#35222=ORIENTED_EDGE ( 'NONE', *, *, #32470, .F. ) ;
#35316=ORIENTED_EDGE ( 'NONE', *, *, #32600, .T. ) ;
#35524=ORIENTED_EDGE ( 'NONE', *, *, #439, .T. ) ;
#35553=CARTESIAN_POINT ( 'NONE',  ( 3.876432148649220366, 11.62356785135076542, -80.65254291642212081 ) ) ;
#35585=EDGE_CURVE ( 'NONE', #37991, #26187, #21723, .T. ) ;
#35687=CYLINDRICAL_SURFACE ( 'NONE', #39353, 0.5000000000000006661 ) ;
#35710=LINE ( 'NONE', #32304, #599 ) ;
#35779=DIRECTION ( 'NONE',  ( 0.000000000000000000, 0.000000000000000000, -1.000000000000000000 ) ) ;
#35858=CARTESIAN_POINT ( 'NONE',  ( 0.000000000000000000, 0.000000000000000000, -80.15254291642212081 ) ) ;
#35924=DIRECTION ( 'NONE',  ( 1.000000000000000000, 0.000000000000000000, 0.000000000000000000 ) ) ;
#36050=EDGE_CURVE ( 'NONE', #24919, #8374, #13321, .T. ) ;
#36051=ORIENTED_EDGE ( 'NONE', *, *, #22999, .F. ) ;
#36060=EDGE_CURVE ( 'NONE', #27278, #19607, #13401, .T. ) ;
#36111=LINE ( 'NONE', #20173, #9161 ) ;
#36113=ADVANCED_FACE ( 'NONE', ( #33777 ), #1238, .T. ) ;
#36116=CARTESIAN_POINT ( 'NONE',  ( 13.27287875805592776, 13.27287875805599704, -80.15254291642212081 ) ) ;
#36145=AXIS2_PLACEMENT_3D ( 'NONE', #17110, #36673, #10722 ) ;
#36255=ORIENTED_EDGE ( 'NONE', *, *, #11401, .T. ) ;
#36259=EDGE_CURVE ( 'NONE', #40461, #18881, #28260, .T. ) ;
#36285=CYLINDRICAL_SURFACE ( 'NONE', #24111, 0.5000000000000000000 ) ;
#36304=CARTESIAN_POINT ( 'NONE',  ( -5.876432148649216813, 13.62356785135076365, -80.65254291642212081 ) ) ;
#36318=EDGE_CURVE ( 'NONE', #18428, #27278, #41202, .T. ) ;
#36354=LINE ( 'NONE', #16589, #26444 ) ;
#36458=EDGE_LOOP ( 'NONE', ( #26679, #37320, #22870, #11202 ) ) ;
#36496=DIRECTION ( 'NONE',  ( -1.000000000000000000, 0.000000000000000000, 0.000000000000000000 ) ) ;
#36531=ORIENTED_EDGE ( 'NONE', *, *, #25282, .T. ) ;
#36615=CYLINDRICAL_SURFACE ( 'NONE', #36929, 0.5000000000000000000 ) ;
#36650=DIRECTION ( 'NONE',  ( 1.000000000000000000, 0.000000000000000000, 0.000000000000000000 ) ) ;
#36673=DIRECTION ( 'NONE',  ( -0.7071067811865491270, 0.7071067811865460184, 0.000000000000000000 ) ) ;
#36685=ORIENTED_EDGE ( 'NONE', *, *, #17603, .T. ) ;
#36731=LINE ( 'NONE', #7593, #16443 ) ;
#36733=DIRECTION ( 'NONE',  ( -0.000000000000000000, -0.000000000000000000, 1.000000000000000000 ) ) ;
#36746=CARTESIAN_POINT ( 'NONE',  ( 5.876432148649220366, 13.62356785135077075, -85.15254291642213502 ) ) ;
#36798=EDGE_CURVE ( 'NONE', #34859, #19379, #12304, .T. ) ;
#36832=VECTOR ( 'NONE', #36733, 1000.000000000000000 ) ;
#36929=AXIS2_PLACEMENT_3D ( 'NONE', #1918, #4703, #27262 ) ;
#36963=EDGE_CURVE ( 'NONE', #15673, #7018, #10598, .T. ) ;
#36965=EDGE_LOOP ( 'NONE', ( #35316, #21201, #6286, #35222 ) ) ;
#36966=EDGE_CURVE ( 'NONE', #3668, #26187, #4832, .T. ) ;
#37071=EDGE_CURVE ( 'NONE', #37786, #19607, #31400, .T. ) ;
#37083=VECTOR ( 'NONE', #31196, 1000.000000000000000 ) ;
#37101=EDGE_CURVE ( 'NONE', #7018, #34634, #37788, .T. ) ;
#37165=VERTEX_POINT ( 'NONE', #28416 ) ;
#37273=DIRECTION ( 'NONE',  ( 0.7071067811865493491, -0.7071067811865456854, -0.000000000000000000 ) ) ;
#37320=ORIENTED_EDGE ( 'NONE', *, *, #21101, .F. ) ;
#37330=CIRCLE ( 'NONE', #18991, 0.5000000000000004441 ) ;
#37356=DIRECTION ( 'NONE',  ( 0.000000000000000000, 0.000000000000000000, -1.000000000000000000 ) ) ;
#37414=CARTESIAN_POINT ( 'NONE',  ( 5.876432148649218590, 13.62356785135076898, -80.35964969760868826 ) ) ;
#37456=LINE ( 'NONE', #41273, #29246 ) ;
#37465=ORIENTED_EDGE ( 'NONE', *, *, #38353, .F. ) ;
#37549=( GEOMETRIC_REPRESENTATION_CONTEXT ( 3 ) GLOBAL_UNCERTAINTY_ASSIGNED_CONTEXT ( ( #13111 ) ) GLOBAL_UNIT_ASSIGNED_CONTEXT ( ( #20024, #451, #7045 ) ) REPRESENTATION_CONTEXT ( 'NONE', 'WORKASPACE' ) );
#37570=ORIENTED_EDGE ( 'NONE', *, *, #13435, .F. ) ;
#37753=ADVANCED_FACE ( 'NONE', ( #10671 ), #36615, .T. ) ;
#37786=VERTEX_POINT ( 'NONE', #1309 ) ;
#37788=LINE ( 'NONE', #22246, #3163 ) ;
#37873=ORIENTED_EDGE ( 'NONE', *, *, #25936, .T. ) ;
#37970=CARTESIAN_POINT ( 'NONE',  ( -3.876432148649211928, 11.62356785135076720, -84.65254291642213502 ) ) ;
#37975=ORIENTED_EDGE ( 'NONE', *, *, #11318, .F. ) ;
#37991=VERTEX_POINT ( 'NONE', #38072 ) ;
#38026=LINE ( 'NONE', #15919, #34846 ) ;
#38043=CARTESIAN_POINT ( 'NONE',  ( -5.876432148649216813, 13.62356785135076365, -80.65254291642212081 ) ) ;
#38072=CARTESIAN_POINT ( 'NONE',  ( 3.876432148649218590, 23.37643214864920438, -80.65254291642212081 ) ) ;
#38130=CARTESIAN_POINT ( 'NONE',  ( -5.376432148649216813, 21.16932536746266535, -80.15254291642212081 ) ) ;
#38239=DIRECTION ( 'NONE',  ( 0.7071067811865469066, 0.7071067811865481278, 0.000000000000000000 ) ) ;
#38240=EDGE_CURVE ( 'NONE', #40136, #18881, #24041, .T. ) ;
#38245=CARTESIAN_POINT ( 'NONE',  ( -3.876432148649213261, 11.62356785135076898, -80.35964969760867405 ) ) ;
#38251=VERTEX_POINT ( 'NONE', #11866 ) ;
#38280=DIRECTION ( 'NONE',  ( 0.000000000000000000, 0.000000000000000000, -1.000000000000000000 ) ) ;
#38302=ORIENTED_EDGE ( 'NONE', *, *, #36798, .T. ) ;
#38353=EDGE_CURVE ( 'NONE', #39500, #4506, #5280, .T. ) ;
#38392=DIRECTION ( 'NONE',  ( 0.7071067811865490160, -0.7071067811865460184, -0.000000000000000000 ) ) ;
#38409=ORIENTED_EDGE ( 'NONE', *, *, #14813, .T. ) ;
#38509=ORIENTED_EDGE ( 'NONE', *, *, #13732, .F. ) ;
#38626=DIRECTION ( 'NONE',  ( 1.000000000000000000, 0.000000000000000000, 0.000000000000000000 ) ) ;
#38638=PLANE ( 'NONE',  #33380 ) ;
#38643=CARTESIAN_POINT ( 'NONE',  ( 3.790645711022319286, 11.83067463253731155, -80.15254291642212081 ) ) ;
#38648=DIRECTION ( 'NONE',  ( -0.000000000000000000, 0.000000000000000000, 1.000000000000000000 ) ) ;
#38683=ORIENTED_EDGE ( 'NONE', *, *, #35585, .T. ) ;
#38710=DIRECTION ( 'NONE',  ( -1.000000000000000000, 0.000000000000000000, 0.000000000000000000 ) ) ;
#38851=LINE ( 'NONE', #41421, #21933 ) ;
#38916=CIRCLE ( 'NONE', #17851, 3.500000000000003997 ) ;
#38963=CARTESIAN_POINT ( 'NONE',  ( -3.500000000000003997, 17.49999999999998934, -80.65254291642212081 ) ) ;
#39051=FACE_BOUND ( 'NONE', #11102, .T. ) ;
#39067=DIRECTION ( 'NONE',  ( 0.000000000000000000, 1.000000000000000000, -0.000000000000000000 ) ) ;
#39084=ORIENTED_EDGE ( 'NONE', *, *, #6984, .F. ) ;
#39086=CARTESIAN_POINT ( 'NONE',  ( -3.876432148649222142, 23.37643214864920438, -80.65254291642212081 ) ) ;
#39137=EDGE_LOOP ( 'NONE', ( #23182, #26892, #25134, #13087 ) ) ;
#39193=CARTESIAN_POINT ( 'NONE',  ( 3.669325367462670240, 22.87643214864920438, -85.15254291642213502 ) ) ;
#39227=ORIENTED_EDGE ( 'NONE', *, *, #13435, .T. ) ;
#39294=DIRECTION ( 'NONE',  ( -0.000000000000000000, 1.000000000000000000, -0.000000000000000000 ) ) ;
#39301=LINE ( 'NONE', #36116, #12132 ) ;
#39324=ORIENTED_EDGE ( 'NONE', *, *, #23680, .F. ) ;
#39333=ADVANCED_FACE ( 'NONE', ( #6492 ), #731, .T. ) ;
#39353=AXIS2_PLACEMENT_3D ( 'NONE', #41869, #38239, #16139 ) ;
#39370=LINE ( 'NONE', #33650, #7026 ) ;
#39376=ADVANCED_FACE ( 'NONE', ( #17112 ), #951, .F. ) ;
#39500=VERTEX_POINT ( 'NONE', #2077 ) ;
#39510=ORIENTED_EDGE ( 'NONE', *, *, #21264, .F. ) ;
#39553=CARTESIAN_POINT ( 'NONE',  ( -3.876432148649222142, 23.37643214864920438, -80.65254291642212081 ) ) ;
#39647=CARTESIAN_POINT ( 'NONE',  ( 0.000000000000000000, 22.87643214864920438, -84.65254291642213502 ) ) ;
#39664=LINE ( 'NONE', #1384, #32 ) ;
#39745=DIRECTION ( 'NONE',  ( 0.000000000000000000, -1.000000000000000000, -0.000000000000000000 ) ) ;
#39940=CARTESIAN_POINT ( 'NONE',  ( -3.876432148649210152, 11.62356785135076542, -80.65254291642212081 ) ) ;
#40036=CARTESIAN_POINT ( 'NONE',  ( -3.669325367462664911, 12.12356785135076542, -85.15254291642213502 ) ) ;
#40136=VERTEX_POINT ( 'NONE', #38963 ) ;
#40148=ORIENTED_EDGE ( 'NONE', *, *, #37101, .F. ) ;
#40258=ORIENTED_EDGE ( 'NONE', *, *, #15462, .T. ) ;
#40365=DIRECTION ( 'NONE',  ( 0.7071067811865469066, 0.7071067811865481278, 0.000000000000000000 ) ) ;
#40391=CARTESIAN_POINT ( 'NONE',  ( 0.000000000000000000, 17.49999999999998934, -80.65254291642212081 ) ) ;
#40442=AXIS2_PLACEMENT_3D ( 'NONE', #11131, #24112, #36650 ) ;
#40449=ORIENTED_EDGE ( 'NONE', *, *, #32600, .F. ) ;
#40452=ORIENTED_EDGE ( 'NONE', *, *, #514, .T. ) ;
#40460=CIRCLE ( 'NONE', #3777, 0.5000000000000004441 ) ;
#40461=VERTEX_POINT ( 'NONE', #19427 ) ;
#40492=VERTEX_POINT ( 'NONE', #16659 ) ;
#40543=ORIENTED_EDGE ( 'NONE', *, *, #41545, .F. ) ;
#40567=DIRECTION ( 'NONE',  ( -0.000000000000000000, 0.000000000000000000, -1.000000000000000000 ) ) ;
#40569=DIRECTION ( 'NONE',  ( -1.000000000000000000, 0.000000000000000000, 0.000000000000000000 ) ) ;
#40592=CARTESIAN_POINT ( 'NONE',  ( -3.876432148649222142, 23.37643214864920438, -85.15254291642213502 ) ) ;
#40622=ADVANCED_BREP_SHAPE_REPRESENTATION ( '', ( #10193, #40442 ), #22097 ) ;
#40640=CARTESIAN_POINT ( 'NONE',  ( 5.876432148649220366, 22.87643214864920438, -80.65254291642212081 ) ) ;
#40644=DIRECTION ( 'NONE',  ( -0.7071067811865456854, -0.7071067811865493491, 0.000000000000000000 ) ) ;
#40649=ORIENTED_EDGE ( 'NONE', *, *, #34759, .F. ) ;
#40708=TOROIDAL_SURFACE ( 'NONE', #22366, 4.000000000000003553, 0.5000000000000000000 ) ;
#40717=DIRECTION ( 'NONE',  ( 0.000000000000000000, 0.000000000000000000, -1.000000000000000000 ) ) ;
#40765=EDGE_CURVE ( 'NONE', #10530, #21607, #17084, .T. ) ;
#40813=ORIENTED_EDGE ( 'NONE', *, *, #22211, .F. ) ;
#40869=DIRECTION ( 'NONE',  ( -1.000000000000000000, 0.000000000000000000, 0.000000000000000000 ) ) ;
#40870=VECTOR ( 'NONE', #29476, 1000.000000000000000 ) ;
#41009=LINE ( 'NONE', #9952, #7059 ) ;
#41086=EDGE_LOOP ( 'NONE', ( #5130, #38302, #2139, #18216 ) ) ;
#41091=ORIENTED_EDGE ( 'NONE', *, *, #36259, .F. ) ;
#41202=LINE ( 'NONE', #5458, #37083 ) ;
#41236=CARTESIAN_POINT ( 'NONE',  ( 5.376432148649220366, 13.83067463253731688, -80.15254291642212081 ) ) ;
#41273=CARTESIAN_POINT ( 'NONE',  ( 5.376432148649220366, 0.000000000000000000, -85.15254291642213502 ) ) ;
#41421=CARTESIAN_POINT ( 'NONE',  ( 5.876432148649222142, 13.62356785135077253, -84.65254291642213502 ) ) ;
#41510=LINE ( 'NONE', #28310, #16521 ) ;
#41545=EDGE_CURVE ( 'NONE', #2455, #3668, #36111, .T. ) ;
#41546=CARTESIAN_POINT ( 'NONE',  ( 5.522878758055947301, 21.02287875805593487, -85.15254291642213502 ) ) ;
#41675=CLOSED_SHELL ( 'NONE', ( #33912, #17360, #14455, #14183, #18722, #1543, #2517, #39376, #6540, #541, #26609, #16401, #3608, #24263, #18572, #3094, #12508, #12312, #29044, #12783, #739, #6082, #25708, #25187, #36113, #39333, #9260, #18495, #9861, #28948, #17917, #37753 ) ) ;
#41835=CARTESIAN_POINT ( 'NONE',  ( 4.000000000000003553, 17.49999999999998934, -80.65254291642212081 ) ) ;
#41852=CARTESIAN_POINT ( 'NONE',  ( 3.876432148649224807, 11.62356785135076898, -80.35964969760867405 ) ) ;
#41864=EDGE_LOOP ( 'NONE', ( #5718, #12778, #16596, #31807 ) ) ;
#41869=CARTESIAN_POINT ( 'NONE',  ( -13.27287875805594375, 13.27287875805592243, -80.65254291642212081 ) ) ;
#41881=VERTEX_POINT ( 'NONE', #16053 ) ;
#41884=VECTOR ( 'NONE', #32079, 1000.000000000000114 ) ;
#42153=COLOUR_RGB('Black',0.12,0.14,0.17);
#42154=FILL_AREA_STYLE_COLOUR('',#42153);
#42155=FILL_AREA_STYLE('',(#42154));
#42156=SURFACE_STYLE_FILL_AREA(#42155);
#42157=SURFACE_SIDE_STYLE('',(#42156));
#42158=SURFACE_STYLE_USAGE(.BOTH.,#42157);
#42159=PRESENTATION_STYLE_ASSIGNMENT((#42158));
ENDSEC;
END-ISO-10303-21;
